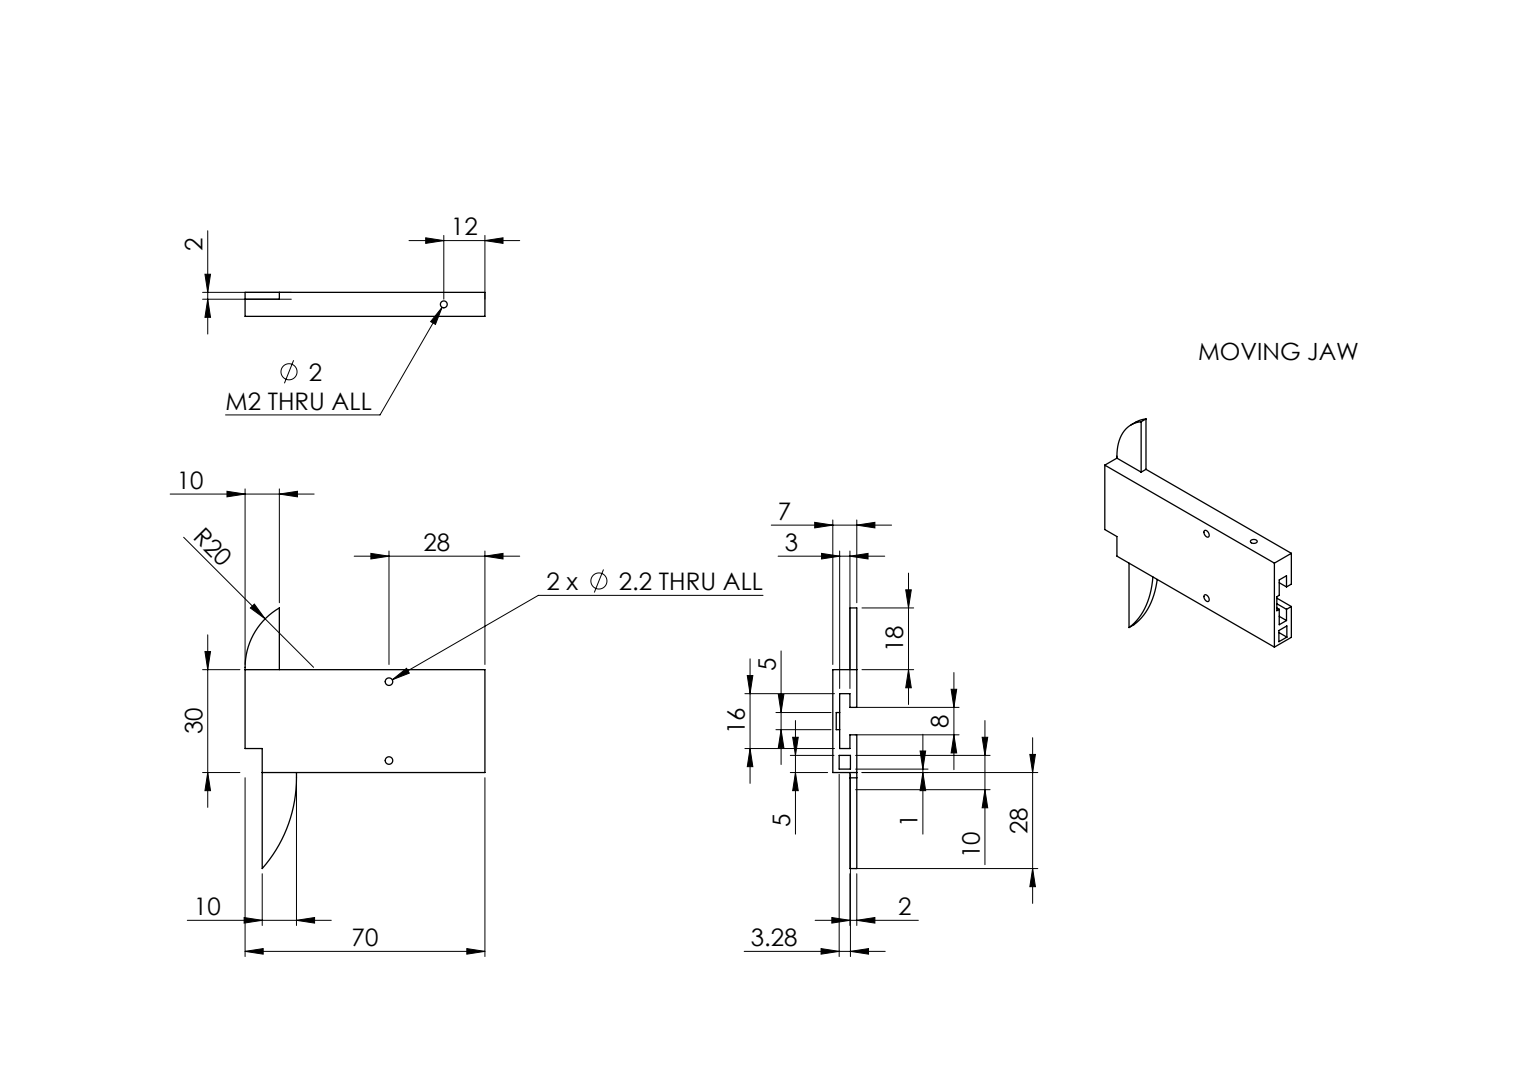
ISO-10303-21;
HEADER;
FILE_DESCRIPTION (('STEP AP214'),
    '1' );
FILE_NAME ('moving jaw.step',
    '2026-10-27T04:40:18',
    ( '' ),
    ( '' ),
    'SwSTEP 2.0',
    'SolidWorks 2026',
    '' );
FILE_SCHEMA (( 'AUTOMOTIVE_DESIGN' ));
ENDSEC;

DATA;
#1=CARTESIAN_POINT ( 'NONE',  ( -49.99998799999998766, -10.00000000000001066, -0.1418111474832477736 ) ) ;
#20=ADVANCED_FACE ( 'NONE', ( #3172 ), #5726, .T. ) ;
#29=ORIENTED_EDGE ( 'NONE', *, *, #855, .F. ) ;
#37=AXIS2_PLACEMENT_3D ( 'NONE', #4538, #3831, #10428 ) ;
#40=VERTEX_POINT ( 'NONE', #7517 ) ;
#41=VERTEX_POINT ( 'NONE', #5843 ) ;
#46=ORIENTED_EDGE ( 'NONE', *, *, #9999, .T. ) ;
#48=PRODUCT ( 'moving jaw', 'moving jaw', '', ( #5785 ) ) ;
#83=SHAPE_REPRESENTATION_RELATIONSHIP ( 'NONE' , 'NONE' ,  #2047, #5753 ) ;
#99=ORIENTED_EDGE ( 'NONE', *, *, #1134, .T. ) ;
#111=LINE ( 'NONE', #735, #8321 ) ;
#115=EDGE_LOOP ( 'NONE', ( #2530, #9133, #537, #4365 ) ) ;
#118=EDGE_CURVE ( 'NONE', #7049, #4198, #6685, .T. ) ;
#125=AXIS2_PLACEMENT_3D ( 'NONE', #8648, #2761, #6933 ) ;
#134=ORIENTED_EDGE ( 'NONE', *, *, #6586, .T. ) ;
#137=FILL_AREA_STYLE ('',( #1868 ) ) ;
#141=EDGE_CURVE ( 'NONE', #5618, #1714, #3939, .T. ) ;
#152=PLANE ( 'NONE',  #5103 ) ;
#159=ORIENTED_EDGE ( 'NONE', *, *, #10440, .T. ) ;
#171=CARTESIAN_POINT ( 'NONE',  ( -77.99999999999998579, 11.49999999999999645, 4.999999999999999112 ) ) ;
#187=CARTESIAN_POINT ( 'NONE',  ( -120.0000000000000000, -4.000000000000019540, -2.000000000000000000 ) ) ;
#201=LINE ( 'NONE', #377, #2655 ) ;
#205=ORIENTED_EDGE ( 'NONE', *, *, #5925, .T. ) ;
#208=LINE ( 'NONE', #3594, #2451 ) ;
#211=VERTEX_POINT ( 'NONE', #6639 ) ;
#214=VECTOR ( 'NONE', #3123, 1000.000000000000000 ) ;
#220=DIRECTION ( 'NONE',  ( -1.000000000000000000, -3.469446951953572774E-16, 0.000000000000000000 ) ) ;
#238=ORIENTED_EDGE ( 'NONE', *, *, #10620, .F. ) ;
#256=( NAMED_UNIT ( * ) SI_UNIT ( $, .STERADIAN. ) SOLID_ANGLE_UNIT ( ) );
#285=FACE_BOUND ( 'NONE', #5927, .T. ) ;
#299=FACE_BOUND ( 'NONE', #9767, .T. ) ;
#306=ORIENTED_EDGE ( 'NONE', *, *, #5403, .T. ) ;
#310=PLANE ( 'NONE',  #5287 ) ;
#324=DIRECTION ( 'NONE',  ( 1.000000000000000000, 2.478176394252581387E-17, 0.000000000000000000 ) ) ;
#330=CARTESIAN_POINT ( 'NONE',  ( -49.99998799999998766, -10.00000000000001066, 5.282956808509874826E-15 ) ) ;
#346=AXIS2_PLACEMENT_3D ( 'NONE', #4920, #5760, #10085 ) ;
#372=DIRECTION ( 'NONE',  ( -1.000000000000000000, 0.000000000000000000, 0.000000000000000000 ) ) ;
#377=CARTESIAN_POINT ( 'NONE',  ( -114.9999999999999289, -7.999999999999998224, -2.000000000000000000 ) ) ;
#378=CYLINDRICAL_SURFACE ( 'NONE', #125, 1.000000000000000888 ) ;
#392=DIRECTION ( 'NONE',  ( 0.000000000000000000, 5.282956808509869699E-16, 1.000000000000000000 ) ) ;
#408=FACE_OUTER_BOUND ( 'NONE', #9322, .T. ) ;
#412=EDGE_CURVE ( 'NONE', #7538, #2208, #10852, .T. ) ;
#417=ORIENTED_EDGE ( 'NONE', *, *, #855, .T. ) ;
#425=AXIS2_PLACEMENT_3D ( 'NONE', #5057, #4070, #1572 ) ;
#426=DIRECTION ( 'NONE',  ( 0.000000000000000000, -0.000000000000000000, -1.000000000000000000 ) ) ;
#430=CARTESIAN_POINT ( 'NONE',  ( -104.9999999999999289, -16.54248688935409106, -2.000000000000000000 ) ) ;
#433=AXIS2_PLACEMENT_3D ( 'NONE', #10103, #729, #1616 ) ;
#448=ORIENTED_EDGE ( 'NONE', *, *, #4377, .F. ) ;
#451=CARTESIAN_POINT ( 'NONE',  ( -49.99999999999998579, -8.000000000000000000, 0.000000000000000000 ) ) ;
#454=DIRECTION ( 'NONE',  ( 1.000000000000000000, 0.000000000000000000, 0.000000000000000000 ) ) ;
#457=CARTESIAN_POINT ( 'NONE',  ( -49.99999999999998579, -2.500000000000000444, 83.15773105863907233 ) ) ;
#460=DIRECTION ( 'NONE',  ( -1.000000000000000000, 0.000000000000000000, 0.000000000000000000 ) ) ;
#462=CARTESIAN_POINT ( 'NONE',  ( -105.0000000000000000, 2.500000000000000000, 3.000000000000000000 ) ) ;
#464=EDGE_LOOP ( 'NONE', ( #3656, #644 ) ) ;
#489=ORIENTED_EDGE ( 'NONE', *, *, #8078, .F. ) ;
#498=LINE ( 'NONE', #8221, #3700 ) ;
#505=VECTOR ( 'NONE', #9411, 1000.000000000000000 ) ;
#512=DIRECTION ( 'NONE',  ( 0.000000000000000000, 1.000000000000000000, 0.000000000000000000 ) ) ;
#518=LINE ( 'NONE', #6516, #873 ) ;
#527=ORIENTED_EDGE ( 'NONE', *, *, #2808, .T. ) ;
#528=CARTESIAN_POINT ( 'NONE',  ( -120.0000000000000000, -4.000000000000019540, 0.000000000000000000 ) ) ;
#536=CIRCLE ( 'NONE', #1421, 40.00000000000000711 ) ;
#537=ORIENTED_EDGE ( 'NONE', *, *, #9340, .T. ) ;
#544=VERTEX_POINT ( 'NONE', #3013 ) ;
#551=VECTOR ( 'NONE', #1388, 1000.000000000000000 ) ;
#558=DIRECTION ( 'NONE',  ( -0.000000000000000000, -0.000000000000000000, -1.000000000000000000 ) ) ;
#566=DIRECTION ( 'NONE',  ( -1.000000000000000000, 0.000000000000000000, 0.000000000000000000 ) ) ;
#570=VERTEX_POINT ( 'NONE', #3901 ) ;
#571=LINE ( 'NONE', #7345, #5302 ) ;
#572=EDGE_CURVE ( 'NONE', #10486, #930, #1997, .T. ) ;
#574=ORIENTED_EDGE ( 'NONE', *, *, #8698, .F. ) ;
#595=CARTESIAN_POINT ( 'NONE',  ( 0.000000000000000000, 0.000000000000000000, 0.000000000000000000 ) ) ;
#596=ORIENTED_EDGE ( 'NONE', *, *, #6504, .F. ) ;
#610=VECTOR ( 'NONE', #6030, 1000.000000000000000 ) ;
#611=CYLINDRICAL_SURFACE ( 'NONE', #4223, 1.099999999999989875 ) ;
#616=CARTESIAN_POINT ( 'NONE',  ( -144.9999999999999147, -16.54248688935410883, -2.000000000000000000 ) ) ;
#624=EDGE_LOOP ( 'NONE', ( #4577, #6804, #1440, #7145 ) ) ;
#631=DIRECTION ( 'NONE',  ( 0.000000000000000000, 0.000000000000000000, -1.000000000000000000 ) ) ;
#639=FACE_OUTER_BOUND ( 'NONE', #8188, .T. ) ;
#643=DIRECTION ( 'NONE',  ( 0.000000000000000000, 0.000000000000000000, -1.000000000000000000 ) ) ;
#644=ORIENTED_EDGE ( 'NONE', *, *, #9959, .F. ) ;
#655=EDGE_LOOP ( 'NONE', ( #7806, #6596, #6590, #7819, #2641, #6040 ) ) ;
#657=EDGE_CURVE ( 'NONE', #5688, #8551, #9953, .T. ) ;
#672=CARTESIAN_POINT ( 'NONE',  ( -76.89999999999999147, -11.50000000000000711, -2.000000000000001332 ) ) ;
#673=DIRECTION ( 'NONE',  ( -3.469446951953572774E-16, 1.000000000000000000, 0.000000000000000000 ) ) ;
#685=ORIENTED_EDGE ( 'NONE', *, *, #10440, .F. ) ;
#699=VECTOR ( 'NONE', #786, 1000.000000000000000 ) ;
#710=VECTOR ( 'NONE', #6574, 1000.000000000000000 ) ;
#716=FACE_OUTER_BOUND ( 'NONE', #7545, .T. ) ;
#719=LINE ( 'NONE', #7497, #9735 ) ;
#726=ORIENTED_EDGE ( 'NONE', *, *, #10589, .F. ) ;
#729=DIRECTION ( 'NONE',  ( 0.000000000000000000, -1.000000000000000000, 0.000000000000000000 ) ) ;
#734=CARTESIAN_POINT ( 'NONE',  ( -120.0000000000000000, 3.999999999999980904, -2.000000000000000000 ) ) ;
#735=CARTESIAN_POINT ( 'NONE',  ( -79.09999999999998010, -11.50000000000000711, -2.000000000000000000 ) ) ;
#761=DIRECTION ( 'NONE',  ( -0.000000000000000000, -0.000000000000000000, 1.000000000000000000 ) ) ;
#785=DIRECTION ( 'NONE',  ( 3.965082230804130220E-16, -1.000000000000000000, -0.000000000000000000 ) ) ;
#786=DIRECTION ( 'NONE',  ( 1.110223024625156540E-15, -1.000000000000000000, -0.000000000000000000 ) ) ;
#795=EDGE_CURVE ( 'NONE', #10821, #9418, #1827, .T. ) ;
#808=LINE ( 'NONE', #4293, #610 ) ;
#824=ORIENTED_EDGE ( 'NONE', *, *, #8252, .F. ) ;
#826=EDGE_CURVE ( 'NONE', #1612, #7049, #10099, .T. ) ;
#851=EDGE_CURVE ( 'NONE', #8859, #6858, #8491, .T. ) ;
#853=CARTESIAN_POINT ( 'NONE',  ( 0.000000000000000000, 2.500000000000000000, 3.000000000000000000 ) ) ;
#855=EDGE_CURVE ( 'NONE', #8551, #10821, #6065, .T. ) ;
#856=VECTOR ( 'NONE', #4422, 1000.000000000000000 ) ;
#859=DIRECTION ( 'NONE',  ( -0.000000000000000000, -0.000000000000000000, -1.000000000000000000 ) ) ;
#862=VECTOR ( 'NONE', #785, 1000.000000000000000 ) ;
#863=ORIENTED_EDGE ( 'NONE', *, *, #9461, .F. ) ;
#865=ORIENTED_EDGE ( 'NONE', *, *, #10184, .F. ) ;
#870=ORIENTED_EDGE ( 'NONE', *, *, #9959, .T. ) ;
#873=VECTOR ( 'NONE', #2385, 1000.000000000000000 ) ;
#877=EDGE_LOOP ( 'NONE', ( #7744, #7640, #7709, #8703, #6978 ) ) ;
#880=ORIENTED_EDGE ( 'NONE', *, *, #964, .F. ) ;
#888=LINE ( 'NONE', #4120, #699 ) ;
#892=CARTESIAN_POINT ( 'NONE',  ( -114.9999999999999289, -7.999999999999998224, 0.000000000000000000 ) ) ;
#914=AXIS2_PLACEMENT_3D ( 'NONE', #7457, #10834, #3218 ) ;
#917=LINE ( 'NONE', #10976, #7086 ) ;
#924=ADVANCED_FACE ( 'NONE', ( #6277 ), #5310, .T. ) ;
#930=VERTEX_POINT ( 'NONE', #6996 ) ;
#960=EDGE_CURVE ( 'NONE', #5520, #211, #7167, .T. ) ;
#964=EDGE_CURVE ( 'NONE', #4466, #8509, #4114, .T. ) ;
#974=CARTESIAN_POINT ( 'NONE',  ( -61.99999999999998579, 14.99999999999998579, 0.5000000000000013323 ) ) ;
#985=EDGE_CURVE ( 'NONE', #4938, #4740, #10490, .T. ) ;
#994=DIRECTION ( 'NONE',  ( 1.000000000000000000, 0.000000000000000000, 0.000000000000000000 ) ) ;
#995=FACE_OUTER_BOUND ( 'NONE', #3796, .T. ) ;
#1027=EDGE_LOOP ( 'NONE', ( #8715, #10682 ) ) ;
#1029=AXIS2_PLACEMENT_3D ( 'NONE', #1383, #4866, #8270 ) ;
#1030=CARTESIAN_POINT ( 'NONE',  ( -109.9999999999999574, 14.99999999999998579, 83.15773105863907233 ) ) ;
#1042=ORIENTED_EDGE ( 'NONE', *, *, #6230, .T. ) ;
#1043=CARTESIAN_POINT ( 'NONE',  ( -49.99999999999998579, 14.99999999999998579, 5.000000000000004441 ) ) ;
#1053=DIRECTION ( 'NONE',  ( -1.000000000000000000, 0.000000000000000000, 0.000000000000000000 ) ) ;
#1080=DIRECTION ( 'NONE',  ( 0.000000000000000000, 1.000000000000000000, 0.000000000000000000 ) ) ;
#1082=FACE_OUTER_BOUND ( 'NONE', #624, .T. ) ;
#1092=ORIENTED_EDGE ( 'NONE', *, *, #9052, .T. ) ;
#1100=EDGE_CURVE ( 'NONE', #3973, #7049, #9351, .T. ) ;
#1107=ADVANCED_FACE ( 'NONE', ( #10181 ), #10074, .F. ) ;
#1112=AXIS2_PLACEMENT_3D ( 'NONE', #9864, #10749, #426 ) ;
#1120=DIRECTION ( 'NONE',  ( -1.000000000000000000, 0.000000000000000000, 0.000000000000000000 ) ) ;
#1134=EDGE_CURVE ( 'NONE', #7831, #4618, #1812, .T. ) ;
#1135=CARTESIAN_POINT ( 'NONE',  ( -105.0000000000000000, -2.500000000000000000, 4.000000000000000000 ) ) ;
#1145=PRESENTATION_STYLE_ASSIGNMENT (( #3639 ) ) ;
#1163=PLANE ( 'NONE',  #7675 ) ;
#1165=DIRECTION ( 'NONE',  ( -1.000000000000000000, 0.000000000000000000, -0.000000000000000000 ) ) ;
#1172=CARTESIAN_POINT ( 'NONE',  ( -61.99999999999998579, 14.99999999999998579, 2.500000000000003109 ) ) ;
#1206=( GEOMETRIC_REPRESENTATION_CONTEXT ( 3 ) GLOBAL_UNCERTAINTY_ASSIGNED_CONTEXT ( ( #10045 ) ) GLOBAL_UNIT_ASSIGNED_CONTEXT ( ( #6328, #8215, #10032 ) ) REPRESENTATION_CONTEXT ( 'NONE', 'WORKASPACE' ) );
#1214=VECTOR ( 'NONE', #9599, 1000.000000000000000 ) ;
#1230=CARTESIAN_POINT ( 'NONE',  ( -149.9999999999999716, 8.000000000000000000, 3.000000000000000000 ) ) ;
#1234=EDGE_LOOP ( 'NONE', ( #6576, #8997, #7608, #685, #8217, #3108 ) ) ;
#1250=AXIS2_PLACEMENT_3D ( 'NONE', #6279, #1542, #9834 ) ;
#1252=DIRECTION ( 'NONE',  ( -1.000000000000000000, 0.000000000000000000, -0.000000000000000000 ) ) ;
#1275=FACE_OUTER_BOUND ( 'NONE', #6489, .T. ) ;
#1285=LINE ( 'NONE', #8070, #10882 ) ;
#1286=DIRECTION ( 'NONE',  ( 1.000000000000000000, 0.000000000000000000, 0.000000000000000000 ) ) ;
#1296=VERTEX_POINT ( 'NONE', #1135 ) ;
#1297=CARTESIAN_POINT ( 'NONE',  ( -77.99999999999998579, -11.50000000000000711, 4.999999999999999112 ) ) ;
#1314=AXIS2_PLACEMENT_3D ( 'NONE', #8865, #8146, #1252 ) ;
#1340=EDGE_LOOP ( 'NONE', ( #238, #5363, #5092, #7261, #4256, #4767, #7735, #1853 ) ) ;
#1355=DIRECTION ( 'NONE',  ( -0.000000000000000000, -0.000000000000000000, 1.000000000000000000 ) ) ;
#1356=FACE_BOUND ( 'NONE', #8492, .T. ) ;
#1357=ORIENTED_EDGE ( 'NONE', *, *, #8744, .F. ) ;
#1362=ORIENTED_EDGE ( 'NONE', *, *, #2808, .F. ) ;
#1370=EDGE_LOOP ( 'NONE', ( #6623, #417, #8003, #8924 ) ) ;
#1380=CARTESIAN_POINT ( 'NONE',  ( -119.9999999999999858, 15.67949192431120053, 0.000000000000000000 ) ) ;
#1383=CARTESIAN_POINT ( 'NONE',  ( -77.99999999999998579, 11.49999999999999645, 4.999999999999999112 ) ) ;
#1388=DIRECTION ( 'NONE',  ( -0.000000000000000000, 1.000000000000000000, -0.000000000000000000 ) ) ;
#1404=AXIS2_PLACEMENT_3D ( 'NONE', #1447, #3009, #5714 ) ;
#1408=ADVANCED_FACE ( 'NONE', ( #3035, #5581 ), #9694, .F. ) ;
#1410=CARTESIAN_POINT ( 'NONE',  ( -120.0000000000000000, -8.000000000000000000, -2.000000000000000000 ) ) ;
#1412=DIRECTION ( 'NONE',  ( -1.000000000000000000, 0.000000000000000000, -0.000000000000000000 ) ) ;
#1415=DIRECTION ( 'NONE',  ( -1.000000000000000000, -0.000000000000000000, -0.000000000000000000 ) ) ;
#1417=CARTESIAN_POINT ( 'NONE',  ( -109.9999999999999574, 14.99999999999998579, -2.000000000000000000 ) ) ;
#1421=AXIS2_PLACEMENT_3D ( 'NONE', #4124, #10850, #4069 ) ;
#1440=ORIENTED_EDGE ( 'NONE', *, *, #5121, .T. ) ;
#1442=ORIENTED_EDGE ( 'NONE', *, *, #8241, .F. ) ;
#1447=CARTESIAN_POINT ( 'NONE',  ( -77.99999999999998579, 11.49999999999999645, -2.000000000000001332 ) ) ;
#1452=VERTEX_POINT ( 'NONE', #9917 ) ;
#1459=CARTESIAN_POINT ( 'NONE',  ( -49.99999999999998579, -15.00000000000001243, 5.000000000000004441 ) ) ;
#1469=LINE ( 'NONE', #9130, #2120 ) ;
#1474=VECTOR ( 'NONE', #2291, 1000.000000000000000 ) ;
#1481=DIRECTION ( 'NONE',  ( -3.965082230804130220E-16, 1.000000000000000000, 0.000000000000000000 ) ) ;
#1490=DIRECTION ( 'NONE',  ( -0.000000000000000000, -0.000000000000000000, -1.000000000000000000 ) ) ;
#1495=EDGE_CURVE ( 'NONE', #3366, #2273, #2351, .T. ) ;
#1499=CARTESIAN_POINT ( 'NONE',  ( -49.99999999999998579, 2.500000000000000000, 4.000000000000000000 ) ) ;
#1500=DIRECTION ( 'NONE',  ( -0.000000000000000000, -0.000000000000000000, -1.000000000000000000 ) ) ;
#1501=CARTESIAN_POINT ( 'NONE',  ( -149.9999999999999716, -8.000000000000000000, 3.000000000000000000 ) ) ;
#1509=CARTESIAN_POINT ( 'NONE',  ( -114.9999999999999289, -15.00000000000001421, 5.000000000000004441 ) ) ;
#1519=ADVANCED_FACE ( 'NONE', ( #639 ), #5792, .F. ) ;
#1542=DIRECTION ( 'NONE',  ( 0.000000000000000000, -1.000000000000000000, 0.000000000000000000 ) ) ;
#1563=VECTOR ( 'NONE', #3177, 1000.000000000000000 ) ;
#1565=DIRECTION ( 'NONE',  ( 1.000000000000000000, -0.000000000000000000, 0.000000000000000000 ) ) ;
#1566=CARTESIAN_POINT ( 'NONE',  ( -114.9999999999999289, -15.00000000000001421, 0.000000000000000000 ) ) ;
#1572=DIRECTION ( 'NONE',  ( 0.000000000000000000, 0.000000000000000000, 1.000000000000000000 ) ) ;
#1577=DIRECTION ( 'NONE',  ( -1.000000000000000000, -3.469446951953572774E-16, 0.000000000000000000 ) ) ;
#1583=DIRECTION ( 'NONE',  ( -1.000000000000000000, 0.000000000000000000, -0.000000000000000000 ) ) ;
#1595=CARTESIAN_POINT ( 'NONE',  ( -114.9999999999999147, -43.00000000000000000, -2.000000000000000000 ) ) ;
#1599=VERTEX_POINT ( 'NONE', #2455 ) ;
#1602=ORIENTED_EDGE ( 'NONE', *, *, #118, .T. ) ;
#1612=VERTEX_POINT ( 'NONE', #4125 ) ;
#1616=DIRECTION ( 'NONE',  ( 0.000000000000000000, 0.000000000000000000, -1.000000000000000000 ) ) ;
#1622=DIRECTION ( 'NONE',  ( 0.000000000000000000, -0.000000000000000000, -1.000000000000000000 ) ) ;
#1623=AXIS2_PLACEMENT_3D ( 'NONE', #9057, #2172, #7494 ) ;
#1644=EDGE_CURVE ( 'NONE', #3802, #570, #6077, .T. ) ;
#1650=AXIS2_PLACEMENT_3D ( 'NONE', #595, #643, #7419 ) ;
#1652=DIRECTION ( 'NONE',  ( 0.000000000000000000, 0.000000000000000000, 1.000000000000000000 ) ) ;
#1657=CARTESIAN_POINT ( 'NONE',  ( -49.99998799999998766, -10.00000000000000888, 3.141811147483251965 ) ) ;
#1664=VECTOR ( 'NONE', #4606, 1000.000000000000000 ) ;
#1694=EDGE_CURVE ( 'NONE', #1612, #1296, #8738, .T. ) ;
#1698=VERTEX_POINT ( 'NONE', #8512 ) ;
#1706=DIRECTION ( 'NONE',  ( 1.000000000000000000, 0.000000000000000000, 0.000000000000000000 ) ) ;
#1714=VERTEX_POINT ( 'NONE', #2682 ) ;
#1725=LINE ( 'NONE', #6950, #10974 ) ;
#1748=EDGE_CURVE ( 'NONE', #570, #3802, #2899, .T. ) ;
#1756=LINE ( 'NONE', #7648, #5474 ) ;
#1758=VECTOR ( 'NONE', #994, 1000.000000000000000 ) ;
#1765=STYLED_ITEM ( 'NONE', ( #1145 ), #5753 ) ;
#1790=CARTESIAN_POINT ( 'NONE',  ( -61.99999999999998579, 14.99999999999998579, 1.500000000000002220 ) ) ;
#1812=CIRCLE ( 'NONE', #7492, 1.000000000000000888 ) ;
#1814=ADVANCED_FACE ( 'NONE', ( #1356, #408 ), #3904, .F. ) ;
#1827=LINE ( 'NONE', #5200, #3582 ) ;
#1828=ORIENTED_EDGE ( 'NONE', *, *, #10681, .F. ) ;
#1829=CARTESIAN_POINT ( 'NONE',  ( -114.9999999999999289, -7.999999999999998224, 5.000000000000004441 ) ) ;
#1831=PRODUCT_DEFINITION_SHAPE ( 'NONE', 'NONE',  #3118 ) ;
#1852=CARTESIAN_POINT ( 'NONE',  ( -120.0000000000000000, -8.000000000000000000, -2.000000000000000000 ) ) ;
#1853=ORIENTED_EDGE ( 'NONE', *, *, #6704, .T. ) ;
#1868=FILL_AREA_STYLE_COLOUR ( '', #6571 ) ;
#1872=LINE ( 'NONE', #5243, #5665 ) ;
#1888=CARTESIAN_POINT ( 'NONE',  ( -49.99998799999998766, -14.00000000000001243, -0.1418111474832477736 ) ) ;
#1918=ORIENTED_EDGE ( 'NONE', *, *, #2411, .F. ) ;
#1923=VECTOR ( 'NONE', #9384, 1000.000000000000000 ) ;
#1934=DIRECTION ( 'NONE',  ( 0.000000000000000000, 0.000000000000000000, -1.000000000000000000 ) ) ;
#1947=CARTESIAN_POINT ( 'NONE',  ( -49.99999999999998579, -14.00000000000001243, -0.1418111474832540464 ) ) ;
#1948=ADVANCED_FACE ( 'NONE', ( #5445 ), #8851, .T. ) ;
#1957=EDGE_LOOP ( 'NONE', ( #596, #5706, #4141, #6991 ) ) ;
#1963=LINE ( 'NONE', #6962, #7655 ) ;
#1970=LINE ( 'NONE', #9577, #10874 ) ;
#1977=EDGE_LOOP ( 'NONE', ( #10642, #6739 ) ) ;
#1987=EDGE_CURVE ( 'NONE', #6146, #3291, #10736, .T. ) ;
#1995=DIRECTION ( 'NONE',  ( 0.000000000000000000, -0.000000000000000000, 1.000000000000000000 ) ) ;
#1997=CIRCLE ( 'NONE', #3066, 1.099999999999989875 ) ;
#2032=ORIENTED_EDGE ( 'NONE', *, *, #5591, .F. ) ;
#2036=ORIENTED_EDGE ( 'NONE', *, *, #4732, .T. ) ;
#2038=CARTESIAN_POINT ( 'NONE',  ( -99.99999999999998579, 15.67949192431120053, -2.000000000000000000 ) ) ;
#2042=EDGE_CURVE ( 'NONE', #10433, #1452, #1970, .T. ) ;
#2044=ORIENTED_EDGE ( 'NONE', *, *, #9484, .T. ) ;
#2047=SHAPE_REPRESENTATION ( 'moving jaw', ( #2307 ), #4948 ) ;
#2053=CARTESIAN_POINT ( 'NONE',  ( -120.0000000000000000, -15.00000000000001421, -2.000000000000000000 ) ) ;
#2054=EDGE_LOOP ( 'NONE', ( #2057, #2218, #8952, #10553 ) ) ;
#2056=EDGE_CURVE ( 'NONE', #3973, #3104, #6857, .T. ) ;
#2057=ORIENTED_EDGE ( 'NONE', *, *, #5007, .F. ) ;
#2061=DIRECTION ( 'NONE',  ( 0.000000000000000000, 1.000000000000000000, 0.000000000000000000 ) ) ;
#2067=DIRECTION ( 'NONE',  ( 0.000000000000000000, -1.000000000000000000, 0.000000000000000000 ) ) ;
#2079=DIRECTION ( 'NONE',  ( -0.000000000000000000, 1.000000000000000000, -0.000000000000000000 ) ) ;
#2090=CARTESIAN_POINT ( 'NONE',  ( -49.99999999999998579, -14.00000000000001243, 3.141811147483255073 ) ) ;
#2091=DIRECTION ( 'NONE',  ( -0.000000000000000000, -0.000000000000000000, -1.000000000000000000 ) ) ;
#2092=ORIENTED_EDGE ( 'NONE', *, *, #9950, .F. ) ;
#2100=EDGE_CURVE ( 'NONE', #4938, #3792, #6020, .T. ) ;
#2109=CARTESIAN_POINT ( 'NONE',  ( -144.9999999999999147, -16.54248688935410883, 0.000000000000000000 ) ) ;
#2110=ORIENTED_EDGE ( 'NONE', *, *, #2887, .F. ) ;
#2120=VECTOR ( 'NONE', #1415, 1000.000000000000000 ) ;
#2140=CARTESIAN_POINT ( 'NONE',  ( -61.99999999999998579, 14.99999999999998579, 1.500000000000002220 ) ) ;
#2171=ORIENTED_EDGE ( 'NONE', *, *, #6545, .T. ) ;
#2172=DIRECTION ( 'NONE',  ( 0.000000000000000000, 0.000000000000000000, -1.000000000000000000 ) ) ;
#2175=DIRECTION ( 'NONE',  ( 0.000000000000000000, 0.000000000000000000, -1.000000000000000000 ) ) ;
#2181=ADVANCED_FACE ( 'NONE', ( #3629 ), #6809, .F. ) ;
#2188=VERTEX_POINT ( 'NONE', #1417 ) ;
#2196=DIRECTION ( 'NONE',  ( 0.000000000000000000, 0.000000000000000000, 1.000000000000000000 ) ) ;
#2204=VERTEX_POINT ( 'NONE', #10463 ) ;
#2208=VERTEX_POINT ( 'NONE', #6251 ) ;
#2210=AXIS2_PLACEMENT_3D ( 'NONE', #2953, #6816, #5073 ) ;
#2218=ORIENTED_EDGE ( 'NONE', *, *, #5229, .F. ) ;
#2233=DIRECTION ( 'NONE',  ( -0.000000000000000000, -0.000000000000000000, -1.000000000000000000 ) ) ;
#2245=PLANE ( 'NONE',  #7427 ) ;
#2248=CARTESIAN_POINT ( 'NONE',  ( -105.0000000000000000, 2.500000000000000000, 4.000000000000000000 ) ) ;
#2258=VERTEX_POINT ( 'NONE', #8094 ) ;
#2273=VERTEX_POINT ( 'NONE', #5629 ) ;
#2275=VECTOR ( 'NONE', #8665, 1000.000000000000000 ) ;
#2283=AXIS2_PLACEMENT_3D ( 'NONE', #8664, #6785, #2501 ) ;
#2291=DIRECTION ( 'NONE',  ( 0.000000000000000000, -1.000000000000000000, 0.000000000000000000 ) ) ;
#2305=LINE ( 'NONE', #3501, #2306 ) ;
#2306=VECTOR ( 'NONE', #7793, 1000.000000000000000 ) ;
#2307=AXIS2_PLACEMENT_3D ( 'NONE', #5193, #3646, #1706 ) ;
#2328=ADVANCED_FACE ( 'NONE', ( #299, #7976 ), #4736, .T. ) ;
#2335=DIRECTION ( 'NONE',  ( -1.000000000000000000, 0.000000000000000000, 0.000000000000000000 ) ) ;
#2341=DIRECTION ( 'NONE',  ( 0.000000000000000000, 0.000000000000000000, -1.000000000000000000 ) ) ;
#2347=FACE_OUTER_BOUND ( 'NONE', #7855, .T. ) ;
#2351=LINE ( 'NONE', #9970, #10146 ) ;
#2352=AXIS2_PLACEMENT_3D ( 'NONE', #10029, #5915, #1583 ) ;
#2366=DIRECTION ( 'NONE',  ( -1.000000000000000000, 0.000000000000000000, 0.000000000000000000 ) ) ;
#2374=ORIENTED_EDGE ( 'NONE', *, *, #5254, .T. ) ;
#2376=VERTEX_POINT ( 'NONE', #672 ) ;
#2379=LINE ( 'NONE', #7496, #9200 ) ;
#2385=DIRECTION ( 'NONE',  ( -0.000000000000000000, -0.000000000000000000, 1.000000000000000000 ) ) ;
#2391=CARTESIAN_POINT ( 'NONE',  ( -49.99999999999998579, -15.00000000000001243, 5.000000000000004441 ) ) ;
#2399=ORIENTED_EDGE ( 'NONE', *, *, #10843, .T. ) ;
#2401=EDGE_CURVE ( 'NONE', #2572, #8685, #3085, .T. ) ;
#2411=EDGE_CURVE ( 'NONE', #8509, #8229, #4059, .T. ) ;
#2418=LINE ( 'NONE', #8374, #4937 ) ;
#2435=LINE ( 'NONE', #6624, #10095 ) ;
#2451=VECTOR ( 'NONE', #6937, 1000.000000000000000 ) ;
#2452=CARTESIAN_POINT ( 'NONE',  ( -105.0000000000000000, 0.000000000000000000, 3.000000000000000000 ) ) ;
#2455=CARTESIAN_POINT ( 'NONE',  ( -120.0000000000000000, 8.000000000000000000, 0.000000000000000000 ) ) ;
#2472=CARTESIAN_POINT ( 'NONE',  ( -61.99999999999998579, -15.00000000000001421, 1.500000000000002220 ) ) ;
#2484=ORIENTED_EDGE ( 'NONE', *, *, #7252, .T. ) ;
#2501=DIRECTION ( 'NONE',  ( 0.000000000000000000, 0.000000000000000000, 1.000000000000000000 ) ) ;
#2510=DIRECTION ( 'NONE',  ( 0.000000000000000000, -1.000000000000000000, 0.000000000000000000 ) ) ;
#2513=CARTESIAN_POINT ( 'NONE',  ( -61.99999999999998579, 14.99999999999998579, 1.500000000000002220 ) ) ;
#2514=CLOSED_SHELL ( 'NONE', ( #5138, #1519, #6235, #7428, #1408, #1814, #2328, #2854, #2804, #7177, #9480, #8967, #9873, #4092, #4117, #3301, #5550, #1107, #1948, #4029, #5963, #6423, #2784, #6008, #4487, #2181, #4923, #4555, #5342, #5724, #924, #10376, #9047, #2947, #5677, #3237, #20, #3957, #7646, #8158, #8848 ) ) ;
#2519=ORIENTED_EDGE ( 'NONE', *, *, #6829, .T. ) ;
#2529=CARTESIAN_POINT ( 'NONE',  ( -49.99999999999998579, -14.00000000000001243, 83.15773105863907233 ) ) ;
#2530=ORIENTED_EDGE ( 'NONE', *, *, #985, .T. ) ;
#2541=ORIENTED_EDGE ( 'NONE', *, *, #10681, .T. ) ;
#2550=DIRECTION ( 'NONE',  ( -0.000000000000000000, -0.000000000000000000, -1.000000000000000000 ) ) ;
#2560=CARTESIAN_POINT ( 'NONE',  ( -49.99999999999998579, -15.00000000000001243, 4.000000000000003553 ) ) ;
#2571=CARTESIAN_POINT ( 'NONE',  ( -61.99999999999998579, 14.99999999999998579, 0.5000000000000013323 ) ) ;
#2572=VERTEX_POINT ( 'NONE', #4262 ) ;
#2587=EDGE_CURVE ( 'NONE', #9263, #2273, #6891, .T. ) ;
#2625=ORIENTED_EDGE ( 'NONE', *, *, #2056, .T. ) ;
#2639=LINE ( 'NONE', #6025, #505 ) ;
#2641=ORIENTED_EDGE ( 'NONE', *, *, #6974, .F. ) ;
#2650=ORIENTED_EDGE ( 'NONE', *, *, #9461, .T. ) ;
#2655=VECTOR ( 'NONE', #8770, 1000.000000000000000 ) ;
#2665=ORIENTED_EDGE ( 'NONE', *, *, #9052, .F. ) ;
#2676=LINE ( 'NONE', #5212, #1758 ) ;
#2682=CARTESIAN_POINT ( 'NONE',  ( -61.99999999999998579, -8.000000000000000000, 0.5000000000000013323 ) ) ;
#2693=EDGE_CURVE ( 'NONE', #4361, #5520, #1285, .T. ) ;
#2705=LINE ( 'NONE', #974, #3898 ) ;
#2707=VECTOR ( 'NONE', #10392, 1000.000000000000000 ) ;
#2726=LINE ( 'NONE', #4435, #7598 ) ;
#2747=DIRECTION ( 'NONE',  ( -1.000000000000000000, -0.000000000000000000, -0.000000000000000000 ) ) ;
#2761=DIRECTION ( 'NONE',  ( -0.000000000000000000, 1.000000000000000000, -0.000000000000000000 ) ) ;
#2765=EDGE_LOOP ( 'NONE', ( #10564, #10658, #6014, #824 ) ) ;
#2774=ORIENTED_EDGE ( 'NONE', *, *, #412, .T. ) ;
#2782=DIRECTION ( 'NONE',  ( 0.000000000000000000, 0.000000000000000000, -1.000000000000000000 ) ) ;
#2784=ADVANCED_FACE ( 'NONE', ( #3780 ), #7228, .T. ) ;
#2788=CARTESIAN_POINT ( 'NONE',  ( 0.000000000000000000, 0.000000000000000000, 5.000000000000000000 ) ) ;
#2804=ADVANCED_FACE ( 'NONE', ( #4714 ), #3062, .F. ) ;
#2808=EDGE_CURVE ( 'NONE', #2208, #10486, #3720, .T. ) ;
#2826=ORIENTED_EDGE ( 'NONE', *, *, #9859, .F. ) ;
#2829=CARTESIAN_POINT ( 'NONE',  ( -49.99999999999998579, 8.000000000000001776, 83.15773105863907233 ) ) ;
#2840=AXIS2_PLACEMENT_3D ( 'NONE', #2788, #7066, #5389 ) ;
#2854=ADVANCED_FACE ( 'NONE', ( #6459, #5607 ), #8177, .F. ) ;
#2865=ORIENTED_EDGE ( 'NONE', *, *, #5787, .F. ) ;
#2884=AXIS2_PLACEMENT_3D ( 'NONE', #4167, #4122, #6532 ) ;
#2887=EDGE_CURVE ( 'NONE', #1698, #2376, #4857, .T. ) ;
#2897=FACE_OUTER_BOUND ( 'NONE', #3419, .T. ) ;
#2899=CIRCLE ( 'NONE', #9104, 1.000000000000000888 ) ;
#2904=PLANE ( 'NONE',  #9212 ) ;
#2907=ORIENTED_EDGE ( 'NONE', *, *, #9894, .T. ) ;
#2925=EDGE_CURVE ( 'NONE', #9418, #5688, #808, .T. ) ;
#2935=DIRECTION ( 'NONE',  ( -0.000000000000000000, -1.000000000000000000, -0.000000000000000000 ) ) ;
#2947=ADVANCED_FACE ( 'NONE', ( #5921 ), #9307, .F. ) ;
#2953=CARTESIAN_POINT ( 'NONE',  ( -120.0000000000000000, -15.00000000000001421, 83.15773105863907233 ) ) ;
#2988=CARTESIAN_POINT ( 'NONE',  ( 0.000000000000000000, -2.500000000000000000, 3.000000000000000000 ) ) ;
#2991=AXIS2_PLACEMENT_3D ( 'NONE', #2140, #2079, #2196 ) ;
#2999=CIRCLE ( 'NONE', #1404, 1.099999999999989875 ) ;
#3009=DIRECTION ( 'NONE',  ( -0.000000000000000000, -0.000000000000000000, -1.000000000000000000 ) ) ;
#3013=CARTESIAN_POINT ( 'NONE',  ( -49.99999999999998579, -2.500000000000000000, 3.000000000000000000 ) ) ;
#3014=ORIENTED_EDGE ( 'NONE', *, *, #10500, .T. ) ;
#3026=ORIENTED_EDGE ( 'NONE', *, *, #1748, .T. ) ;
#3035=FACE_OUTER_BOUND ( 'NONE', #1234, .T. ) ;
#3062=PLANE ( 'NONE',  #6813 ) ;
#3066=AXIS2_PLACEMENT_3D ( 'NONE', #5324, #2233, #2335 ) ;
#3070=LINE ( 'NONE', #9849, #4080 ) ;
#3073=DIRECTION ( 'NONE',  ( -1.000000000000000000, 0.000000000000000000, 0.000000000000000000 ) ) ;
#3081=PLANE ( 'NONE',  #6384 ) ;
#3085=CIRCLE ( 'NONE', #433, 1.000000000000000888 ) ;
#3095=FACE_OUTER_BOUND ( 'NONE', #10378, .T. ) ;
#3100=ORIENTED_EDGE ( 'NONE', *, *, #5058, .F. ) ;
#3104=VERTEX_POINT ( 'NONE', #1499 ) ;
#3108=ORIENTED_EDGE ( 'NONE', *, *, #5529, .T. ) ;
#3118=PRODUCT_DEFINITION ( 'UNKNOWN', '', #7460, #8348 ) ;
#3120=CARTESIAN_POINT ( 'NONE',  ( -49.99999999999998579, 8.000000000000000000, 3.000000000000000000 ) ) ;
#3123=DIRECTION ( 'NONE',  ( 0.000000000000000000, 0.000000000000000000, -1.000000000000000000 ) ) ;
#3141=CARTESIAN_POINT ( 'NONE',  ( -114.9999999999999289, -7.999999999999998224, -2.000000000000000000 ) ) ;
#3152=VERTEX_POINT ( 'NONE', #6199 ) ;
#3157=LINE ( 'NONE', #8320, #551 ) ;
#3167=EDGE_CURVE ( 'NONE', #8229, #5900, #9987, .T. ) ;
#3172=FACE_OUTER_BOUND ( 'NONE', #10185, .T. ) ;
#3177=DIRECTION ( 'NONE',  ( 1.000000000000000000, 0.000000000000000000, 0.000000000000000000 ) ) ;
#3209=ORIENTED_EDGE ( 'NONE', *, *, #5754, .T. ) ;
#3218=DIRECTION ( 'NONE',  ( 1.000000000000000000, 0.000000000000000000, -0.000000000000000000 ) ) ;
#3224=FACE_BOUND ( 'NONE', #1027, .T. ) ;
#3232=ORIENTED_EDGE ( 'NONE', *, *, #7753, .F. ) ;
#3237=ADVANCED_FACE ( 'NONE', ( #4579 ), #5237, .T. ) ;
#3257=ORIENTED_EDGE ( 'NONE', *, *, #5403, .F. ) ;
#3262=ORIENTED_EDGE ( 'NONE', *, *, #7252, .F. ) ;
#3284=CYLINDRICAL_SURFACE ( 'NONE', #7591, 1.099999999999989875 ) ;
#3291=VERTEX_POINT ( 'NONE', #4026 ) ;
#3297=CARTESIAN_POINT ( 'NONE',  ( -61.99999999999998579, -15.00000000000001421, 2.500000000000003109 ) ) ;
#3301=ADVANCED_FACE ( 'NONE', ( #3095 ), #9817, .T. ) ;
#3366=VERTEX_POINT ( 'NONE', #4907 ) ;
#3375=DIRECTION ( 'NONE',  ( -0.000000000000000000, -0.000000000000000000, -1.000000000000000000 ) ) ;
#3377=FACE_OUTER_BOUND ( 'NONE', #9807, .T. ) ;
#3396=ORIENTED_EDGE ( 'NONE', *, *, #1100, .T. ) ;
#3419=EDGE_LOOP ( 'NONE', ( #2541, #10410, #7823, #7330 ) ) ;
#3421=DIRECTION ( 'NONE',  ( -1.000000000000000000, 0.000000000000000000, 0.000000000000000000 ) ) ;
#3431=VERTEX_POINT ( 'NONE', #9295 ) ;
#3443=DIRECTION ( 'NONE',  ( -0.000000000000000000, -0.000000000000000000, 1.000000000000000000 ) ) ;
#3484=ORIENTED_EDGE ( 'NONE', *, *, #5576, .F. ) ;
#3495=LINE ( 'NONE', #8616, #6560 ) ;
#3501=CARTESIAN_POINT ( 'NONE',  ( -120.0000000000000000, 8.000000000000000000, 83.15773105863907233 ) ) ;
#3515=ORIENTED_EDGE ( 'NONE', *, *, #1495, .T. ) ;
#3523=ORIENTED_EDGE ( 'NONE', *, *, #9098, .T. ) ;
#3527=DIRECTION ( 'NONE',  ( -0.000000000000000000, -0.000000000000000000, -1.000000000000000000 ) ) ;
#3531=CIRCLE ( 'NONE', #10263, 1.000000000000000888 ) ;
#3558=CARTESIAN_POINT ( 'NONE',  ( -114.9999999999999289, -7.999999999999998224, -2.000000000000000000 ) ) ;
#3582=VECTOR ( 'NONE', #8437, 1000.000000000000000 ) ;
#3585=VERTEX_POINT ( 'NONE', #1509 ) ;
#3586=CARTESIAN_POINT ( 'NONE',  ( -61.99999999999998579, -15.00000000000001421, 1.500000000000002220 ) ) ;
#3592=EDGE_CURVE ( 'NONE', #9418, #5520, #6577, .T. ) ;
#3594=CARTESIAN_POINT ( 'NONE',  ( -120.0000000000000000, 3.999999999999980904, -2.000000000000000000 ) ) ;
#3607=EDGE_CURVE ( 'NONE', #2376, #1698, #4827, .T. ) ;
#3608=CARTESIAN_POINT ( 'NONE',  ( -104.9999999999999147, -15.00000000000001421, 0.000000000000000000 ) ) ;
#3617=EDGE_CURVE ( 'NONE', #3964, #8912, #9902, .T. ) ;
#3623=ORIENTED_EDGE ( 'NONE', *, *, #10813, .T. ) ;
#3629=FACE_OUTER_BOUND ( 'NONE', #2765, .T. ) ;
#3639=SURFACE_STYLE_USAGE ( .BOTH. , #6203 ) ;
#3646=DIRECTION ( 'NONE',  ( 0.000000000000000000, 0.000000000000000000, 1.000000000000000000 ) ) ;
#3656=ORIENTED_EDGE ( 'NONE', *, *, #141, .F. ) ;
#3660=CARTESIAN_POINT ( 'NONE',  ( -149.9999999999999716, -8.000000000000000000, 3.000000000000000000 ) ) ;
#3665=DIRECTION ( 'NONE',  ( 0.000000000000000000, -0.000000000000000000, -1.000000000000000000 ) ) ;
#3667=DIRECTION ( 'NONE',  ( -0.000000000000000000, -0.000000000000000000, -1.000000000000000000 ) ) ;
#3669=FACE_OUTER_BOUND ( 'NONE', #655, .T. ) ;
#3676=FACE_OUTER_BOUND ( 'NONE', #1957, .T. ) ;
#3696=AXIS2_PLACEMENT_3D ( 'NONE', #3838, #2175, #10609 ) ;
#3700=VECTOR ( 'NONE', #6450, 1000.000000000000000 ) ;
#3706=EDGE_LOOP ( 'NONE', ( #8583, #4737, #2374, #3623 ) ) ;
#3720=LINE ( 'NONE', #8122, #1664 ) ;
#3729=LINE ( 'NONE', #1172, #10253 ) ;
#3775=DIRECTION ( 'NONE',  ( 1.000000000000000000, -0.000000000000000000, 0.000000000000000000 ) ) ;
#3780=FACE_OUTER_BOUND ( 'NONE', #10079, .T. ) ;
#3783=AXIS2_PLACEMENT_3D ( 'NONE', #2513, #6689, #10851 ) ;
#3788=PLANE ( 'NONE',  #9928 ) ;
#3792=VERTEX_POINT ( 'NONE', #4157 ) ;
#3795=VECTOR ( 'NONE', #4515, 1000.000000000000000 ) ;
#3796=EDGE_LOOP ( 'NONE', ( #2519, #2032, #2907, #2044 ) ) ;
#3802=VERTEX_POINT ( 'NONE', #4366 ) ;
#3831=DIRECTION ( 'NONE',  ( 0.000000000000000000, -0.000000000000000000, 1.000000000000000000 ) ) ;
#3838=CARTESIAN_POINT ( 'NONE',  ( 0.000000000000000000, 0.000000000000000000, 4.000000000000000000 ) ) ;
#3847=UNCERTAINTY_MEASURE_WITH_UNIT (LENGTH_MEASURE( 1.000000000000000082E-05 ), #4408, 'distance_accuracy_value', 'NONE');
#3855=ORIENTED_EDGE ( 'NONE', *, *, #6412, .T. ) ;
#3887=ORIENTED_EDGE ( 'NONE', *, *, #2925, .F. ) ;
#3888=CARTESIAN_POINT ( 'NONE',  ( -49.99999999999998579, -10.00000000000000888, -0.1418111474832519925 ) ) ;
#3890=VECTOR ( 'NONE', #4949, 1000.000000000000000 ) ;
#3898=VECTOR ( 'NONE', #6147, 1000.000000000000000 ) ;
#3901=CARTESIAN_POINT ( 'NONE',  ( -61.99999999999998579, 14.99999999999998579, 2.500000000000003109 ) ) ;
#3904=PLANE ( 'NONE',  #7164 ) ;
#3924=EDGE_LOOP ( 'NONE', ( #9884, #7845, #4646, #7601 ) ) ;
#3933=ORIENTED_EDGE ( 'NONE', *, *, #10027, .T. ) ;
#3936=DIRECTION ( 'NONE',  ( -1.000000000000000000, 0.000000000000000000, 0.000000000000000000 ) ) ;
#3939=CIRCLE ( 'NONE', #2884, 1.000000000000000888 ) ;
#3941=EDGE_LOOP ( 'NONE', ( #5298, #5003, #7576, #5126, #9431, #6674, #5871, #3855 ) ) ;
#3954=LINE ( 'NONE', #8285, #4605 ) ;
#3955=DIRECTION ( 'NONE',  ( -0.000000000000000000, 1.000000000000000000, 0.000000000000000000 ) ) ;
#3957=ADVANCED_FACE ( 'NONE', ( #5257 ), #1163, .F. ) ;
#3964=VERTEX_POINT ( 'NONE', #1043 ) ;
#3969=PLANE ( 'NONE',  #5656 ) ;
#3973=VERTEX_POINT ( 'NONE', #9783 ) ;
#3994=VERTEX_POINT ( 'NONE', #451 ) ;
#3998=FACE_OUTER_BOUND ( 'NONE', #3941, .T. ) ;
#4003=DIRECTION ( 'NONE',  ( 3.965082230804130220E-16, -1.000000000000000000, -0.000000000000000000 ) ) ;
#4006=ORIENTED_EDGE ( 'NONE', *, *, #412, .F. ) ;
#4010=LINE ( 'NONE', #9019, #4752 ) ;
#4026=CARTESIAN_POINT ( 'NONE',  ( -120.0000000000000000, 8.000000000000000000, 3.000000000000000000 ) ) ;
#4029=ADVANCED_FACE ( 'NONE', ( #6563 ), #6506, .T. ) ;
#4036=ORIENTED_EDGE ( 'NONE', *, *, #2056, .F. ) ;
#4054=VERTEX_POINT ( 'NONE', #8120 ) ;
#4059=LINE ( 'NONE', #7459, #6627 ) ;
#4069=DIRECTION ( 'NONE',  ( -1.000000000000000000, 0.000000000000000000, 0.000000000000000000 ) ) ;
#4070=DIRECTION ( 'NONE',  ( -0.000000000000000000, 1.000000000000000000, -0.000000000000000000 ) ) ;
#4080=VECTOR ( 'NONE', #4780, 1000.000000000000000 ) ;
#4083=ORIENTED_EDGE ( 'NONE', *, *, #7073, .F. ) ;
#4092=ADVANCED_FACE ( 'NONE', ( #7390 ), #10725, .T. ) ;
#4096=ORIENTED_EDGE ( 'NONE', *, *, #960, .T. ) ;
#4100=DIRECTION ( 'NONE',  ( 0.000000000000000000, -0.000000000000000000, 1.000000000000000000 ) ) ;
#4114=CIRCLE ( 'NONE', #37, 20.00000000000000355 ) ;
#4117=ADVANCED_FACE ( 'NONE', ( #716 ), #10877, .F. ) ;
#4118=CARTESIAN_POINT ( 'NONE',  ( -114.9999999999999147, -43.00000000000000000, -2.000000000000000000 ) ) ;
#4120=CARTESIAN_POINT ( 'NONE',  ( -119.9999999999999716, 8.000000000000001776, 0.000000000000000000 ) ) ;
#4122=DIRECTION ( 'NONE',  ( 0.000000000000000000, 1.000000000000000000, 0.000000000000000000 ) ) ;
#4124=CARTESIAN_POINT ( 'NONE',  ( -144.9999999999999147, -16.54248688935410883, -2.000000000000000000 ) ) ;
#4125=CARTESIAN_POINT ( 'NONE',  ( -105.0000000000000000, 2.500000000000000000, 4.000000000000000000 ) ) ;
#4141=ORIENTED_EDGE ( 'NONE', *, *, #6023, .T. ) ;
#4155=CARTESIAN_POINT ( 'NONE',  ( -120.0000000000000000, 14.99999999999998579, 5.000000000000004441 ) ) ;
#4157=CARTESIAN_POINT ( 'NONE',  ( -120.0000000000000000, -4.000000000000019540, 0.000000000000000000 ) ) ;
#4160=CARTESIAN_POINT ( 'NONE',  ( -120.0000000000000000, -4.000000000000019540, -2.000000000000000000 ) ) ;
#4167=CARTESIAN_POINT ( 'NONE',  ( -61.99999999999998579, -8.000000000000000000, 1.500000000000002220 ) ) ;
#4180=EDGE_LOOP ( 'NONE', ( #1442, #7293, #5341, #7707 ) ) ;
#4193=LINE ( 'NONE', #1657, #7636 ) ;
#4198=VERTEX_POINT ( 'NONE', #7812 ) ;
#4223=AXIS2_PLACEMENT_3D ( 'NONE', #8062, #558, #3936 ) ;
#4236=CARTESIAN_POINT ( 'NONE',  ( -120.0000000000000000, 14.99999999999998579, 5.000000000000004441 ) ) ;
#4250=ORIENTED_EDGE ( 'NONE', *, *, #7867, .F. ) ;
#4256=ORIENTED_EDGE ( 'NONE', *, *, #9844, .F. ) ;
#4262=CARTESIAN_POINT ( 'NONE',  ( -61.99999999999998579, 8.000000000000000000, 2.500000000000003109 ) ) ;
#4293=CARTESIAN_POINT ( 'NONE',  ( -120.0000000000000000, -15.00000000000001421, 0.000000000000000000 ) ) ;
#4300=ORIENTED_EDGE ( 'NONE', *, *, #2587, .F. ) ;
#4308=AXIS2_PLACEMENT_3D ( 'NONE', #8589, #859, #4875 ) ;
#4312=LINE ( 'NONE', #1829, #8513 ) ;
#4337=CARTESIAN_POINT ( 'NONE',  ( 0.000000000000000000, 0.000000000000000000, 0.000000000000000000 ) ) ;
#4347=CARTESIAN_POINT ( 'NONE',  ( -49.99999999999998579, 3.999999999999980904, 0.000000000000000000 ) ) ;
#4361=VERTEX_POINT ( 'NONE', #430 ) ;
#4365=ORIENTED_EDGE ( 'NONE', *, *, #2100, .F. ) ;
#4366=CARTESIAN_POINT ( 'NONE',  ( -61.99999999999998579, 14.99999999999998579, 0.5000000000000013323 ) ) ;
#4374=LINE ( 'NONE', #457, #6002 ) ;
#4377=EDGE_CURVE ( 'NONE', #8566, #7983, #10470, .T. ) ;
#4380=LINE ( 'NONE', #3558, #8498 ) ;
#4393=CARTESIAN_POINT ( 'NONE',  ( -49.99999999999998579, 2.500000000000000444, 83.15773105863907233 ) ) ;
#4408=( LENGTH_UNIT ( ) NAMED_UNIT ( * ) SI_UNIT ( .MILLI., .METRE. ) );
#4416=VECTOR ( 'NONE', #6796, 1000.000000000000000 ) ;
#4422=DIRECTION ( 'NONE',  ( 0.000000000000000000, 1.000000000000000000, 0.000000000000000000 ) ) ;
#4428=ORIENTED_EDGE ( 'NONE', *, *, #7372, .T. ) ;
#4435=CARTESIAN_POINT ( 'NONE',  ( -114.9999999999999289, -7.999999999999998224, -2.000000000000000000 ) ) ;
#4436=LINE ( 'NONE', #5497, #7776 ) ;
#4446=EDGE_CURVE ( 'NONE', #9263, #7983, #6259, .T. ) ;
#4454=VECTOR ( 'NONE', #10396, 1000.000000000000000 ) ;
#4460=ORIENTED_EDGE ( 'NONE', *, *, #1987, .T. ) ;
#4466=VERTEX_POINT ( 'NONE', #4576 ) ;
#4470=DIRECTION ( 'NONE',  ( 1.000000000000000000, 0.000000000000000000, 0.000000000000000000 ) ) ;
#4487=ADVANCED_FACE ( 'NONE', ( #4745 ), #6488, .F. ) ;
#4498=DIRECTION ( 'NONE',  ( 0.000000000000000000, 1.000000000000000000, 0.000000000000000000 ) ) ;
#4515=DIRECTION ( 'NONE',  ( 0.000000000000000000, 0.000000000000000000, 1.000000000000000000 ) ) ;
#4516=ORIENTED_EDGE ( 'NONE', *, *, #5254, .F. ) ;
#4538=CARTESIAN_POINT ( 'NONE',  ( -99.99999999999998579, 15.67949192431120053, 0.000000000000000000 ) ) ;
#4539=VERTEX_POINT ( 'NONE', #8260 ) ;
#4540=CARTESIAN_POINT ( 'NONE',  ( -49.99999999999998579, -8.000000000000000000, 3.000000000000000000 ) ) ;
#4544=CARTESIAN_POINT ( 'NONE',  ( -120.0000000000000000, -15.00000000000001421, 83.15773105863907233 ) ) ;
#4555=ADVANCED_FACE ( 'NONE', ( #8303 ), #5693, .F. ) ;
#4576=CARTESIAN_POINT ( 'NONE',  ( -109.9999999999999289, 33.00000000000000711, 0.000000000000000000 ) ) ;
#4577=ORIENTED_EDGE ( 'NONE', *, *, #826, .F. ) ;
#4579=FACE_OUTER_BOUND ( 'NONE', #3924, .T. ) ;
#4585=VERTEX_POINT ( 'NONE', #6747 ) ;
#4593=ORIENTED_EDGE ( 'NONE', *, *, #5320, .F. ) ;
#4596=LINE ( 'NONE', #8000, #856 ) ;
#4605=VECTOR ( 'NONE', #10887, 1000.000000000000000 ) ;
#4606=DIRECTION ( 'NONE',  ( -0.000000000000000000, -0.000000000000000000, -1.000000000000000000 ) ) ;
#4618=VERTEX_POINT ( 'NONE', #3297 ) ;
#4621=DIRECTION ( 'NONE',  ( 0.000000000000000000, 0.000000000000000000, -1.000000000000000000 ) ) ;
#4626=VERTEX_POINT ( 'NONE', #8461 ) ;
#4646=ORIENTED_EDGE ( 'NONE', *, *, #2587, .T. ) ;
#4654=DIRECTION ( 'NONE',  ( 0.000000000000000000, -1.000000000000000000, 0.000000000000000000 ) ) ;
#4665=DIRECTION ( 'NONE',  ( -0.000000000000000000, 1.000000000000000000, 0.000000000000000000 ) ) ;
#4707=EDGE_CURVE ( 'NONE', #3104, #1612, #1963, .T. ) ;
#4709=DIRECTION ( 'NONE',  ( -0.000000000000000000, -1.000000000000000000, -0.000000000000000000 ) ) ;
#4714=FACE_OUTER_BOUND ( 'NONE', #115, .T. ) ;
#4730=LINE ( 'NONE', #528, #1563 ) ;
#4732=EDGE_CURVE ( 'NONE', #8685, #3802, #7799, .T. ) ;
#4736=PLANE ( 'NONE',  #1314 ) ;
#4737=ORIENTED_EDGE ( 'NONE', *, *, #10261, .T. ) ;
#4740=VERTEX_POINT ( 'NONE', #1852 ) ;
#4745=FACE_OUTER_BOUND ( 'NONE', #877, .T. ) ;
#4752=VECTOR ( 'NONE', #10055, 1000.000000000000000 ) ;
#4760=VECTOR ( 'NONE', #1490, 1000.000000000000000 ) ;
#4767=ORIENTED_EDGE ( 'NONE', *, *, #960, .F. ) ;
#4768=DIRECTION ( 'NONE',  ( 0.000000000000000000, 0.000000000000000000, -1.000000000000000000 ) ) ;
#4780=DIRECTION ( 'NONE',  ( -1.000000000000000000, -0.000000000000000000, -0.000000000000000000 ) ) ;
#4815=VECTOR ( 'NONE', #2091, 1000.000000000000000 ) ;
#4819=EDGE_LOOP ( 'NONE', ( #134, #99 ) ) ;
#4827=CIRCLE ( 'NONE', #7500, 1.099999999999989875 ) ;
#4857=CIRCLE ( 'NONE', #10720, 1.099999999999989875 ) ;
#4866=DIRECTION ( 'NONE',  ( -0.000000000000000000, -0.000000000000000000, -1.000000000000000000 ) ) ;
#4870=CARTESIAN_POINT ( 'NONE',  ( -49.99999999999998579, -15.00000000000001243, 0.000000000000000000 ) ) ;
#4875=DIRECTION ( 'NONE',  ( -1.000000000000000000, 0.000000000000000000, 0.000000000000000000 ) ) ;
#4907=CARTESIAN_POINT ( 'NONE',  ( -57.99999999999998579, -14.00000000000001243, 3.141811147483251965 ) ) ;
#4920=CARTESIAN_POINT ( 'NONE',  ( -120.0000000000000000, 3.999999999999980904, -2.000000000000000000 ) ) ;
#4923=ADVANCED_FACE ( 'NONE', ( #5835 ), #8346, .F. ) ;
#4929=DIRECTION ( 'NONE',  ( -1.000000000000000000, -3.965082230804130220E-16, 0.000000000000000000 ) ) ;
#4932=VECTOR ( 'NONE', #1286, 1000.000000000000000 ) ;
#4937=VECTOR ( 'NONE', #761, 1000.000000000000000 ) ;
#4938=VERTEX_POINT ( 'NONE', #4160 ) ;
#4948=( GEOMETRIC_REPRESENTATION_CONTEXT ( 3 ) GLOBAL_UNCERTAINTY_ASSIGNED_CONTEXT ( ( #8082 ) ) GLOBAL_UNIT_ASSIGNED_CONTEXT ( ( #7930, #7704, #256 ) ) REPRESENTATION_CONTEXT ( 'NONE', 'WORKASPACE' ) );
#4949=DIRECTION ( 'NONE',  ( 0.000000000000000000, 1.000000000000000000, -0.000000000000000000 ) ) ;
#4962=VERTEX_POINT ( 'NONE', #5780 ) ;
#4967=CARTESIAN_POINT ( 'NONE',  ( -105.0000000000000000, 2.500000000000000000, 4.000000000000000000 ) ) ;
#4974=PLANE ( 'NONE',  #346 ) ;
#4983=CARTESIAN_POINT ( 'NONE',  ( -114.9999999999999147, -43.00000000000000000, -2.000000000000000000 ) ) ;
#4993=CARTESIAN_POINT ( 'NONE',  ( -114.9999999999999289, -7.999999999999998224, -2.000000000000000000 ) ) ;
#4995=AXIS2_PLACEMENT_3D ( 'NONE', #2109, #7890, #8002 ) ;
#5003=ORIENTED_EDGE ( 'NONE', *, *, #7226, .T. ) ;
#5007=EDGE_CURVE ( 'NONE', #4740, #8859, #6523, .T. ) ;
#5057=CARTESIAN_POINT ( 'NONE',  ( -61.99999999999998579, 14.99999999999998579, 1.500000000000002220 ) ) ;
#5058=EDGE_CURVE ( 'NONE', #7983, #2258, #5151, .T. ) ;
#5068=EDGE_LOOP ( 'NONE', ( #10141, #3484, #5649, #7977 ) ) ;
#5073=DIRECTION ( 'NONE',  ( -1.000000000000000000, -2.478176394252581696E-17, 0.000000000000000000 ) ) ;
#5092=ORIENTED_EDGE ( 'NONE', *, *, #985, .F. ) ;
#5103=AXIS2_PLACEMENT_3D ( 'NONE', #6155, #9540, #1934 ) ;
#5105=ORIENTED_EDGE ( 'NONE', *, *, #5807, .T. ) ;
#5107=CARTESIAN_POINT ( 'NONE',  ( -105.0000000000000000, -2.500000000000000000, 4.000000000000000000 ) ) ;
#5120=DIRECTION ( 'NONE',  ( -2.478176394252581696E-17, 1.000000000000000000, 0.000000000000000000 ) ) ;
#5121=EDGE_CURVE ( 'NONE', #1296, #4198, #8555, .T. ) ;
#5126=ORIENTED_EDGE ( 'NONE', *, *, #6868, .F. ) ;
#5129=( NAMED_UNIT ( * ) PLANE_ANGLE_UNIT ( ) SI_UNIT ( $, .RADIAN. ) );
#5138=ADVANCED_FACE ( 'NONE', ( #7836 ), #7781, .F. ) ;
#5151=LINE ( 'NONE', #1, #9368 ) ;
#5155=LINE ( 'NONE', #10212, #9041 ) ;
#5160=CARTESIAN_POINT ( 'NONE',  ( -114.9999999999999289, -8.000000000000000000, 3.000000000000000000 ) ) ;
#5193=CARTESIAN_POINT ( 'NONE',  ( 0.000000000000000000, 0.000000000000000000, 0.000000000000000000 ) ) ;
#5198=EDGE_CURVE ( 'NONE', #3585, #4054, #10207, .T. ) ;
#5200=CARTESIAN_POINT ( 'NONE',  ( -104.9999999999999289, -7.999999999999994671, 0.000000000000000000 ) ) ;
#5203=DIRECTION ( 'NONE',  ( -1.000000000000000000, 0.000000000000000000, 0.000000000000000000 ) ) ;
#5204=EDGE_LOOP ( 'NONE', ( #3100, #448, #10962, #10666 ) ) ;
#5208=DIRECTION ( 'NONE',  ( -0.000000000000000000, -0.000000000000000000, -1.000000000000000000 ) ) ;
#5212=CARTESIAN_POINT ( 'NONE',  ( -120.0000000000000000, -4.000000000000019540, -2.000000000000000000 ) ) ;
#5229=EDGE_CURVE ( 'NONE', #4626, #4740, #2726, .T. ) ;
#5237=PLANE ( 'NONE',  #5549 ) ;
#5243=CARTESIAN_POINT ( 'NONE',  ( -76.89999999999999147, -11.50000000000000711, -2.000000000000000000 ) ) ;
#5247=VERTEX_POINT ( 'NONE', #6165 ) ;
#5254=EDGE_CURVE ( 'NONE', #6924, #7749, #8010, .T. ) ;
#5255=VECTOR ( 'NONE', #5418, 1000.000000000000000 ) ;
#5257=FACE_OUTER_BOUND ( 'NONE', #5204, .T. ) ;
#5260=CARTESIAN_POINT ( 'NONE',  ( -105.0000000000000000, -2.500000000000000000, 4.000000000000000000 ) ) ;
#5261=CARTESIAN_POINT ( 'NONE',  ( -104.9999999999999289, -16.54248688935409106, -2.000000000000000000 ) ) ;
#5287=AXIS2_PLACEMENT_3D ( 'NONE', #5352, #4470, #7817 ) ;
#5298=ORIENTED_EDGE ( 'NONE', *, *, #657, .F. ) ;
#5300=DIRECTION ( 'NONE',  ( -0.000000000000000000, -0.000000000000000000, -1.000000000000000000 ) ) ;
#5302=VECTOR ( 'NONE', #10735, 1000.000000000000000 ) ;
#5310=PLANE ( 'NONE',  #6957 ) ;
#5316=LINE ( 'NONE', #10437, #6895 ) ;
#5317=CARTESIAN_POINT ( 'NONE',  ( -120.0000000000000000, -15.00000000000001421, 5.000000000000004441 ) ) ;
#5320=EDGE_CURVE ( 'NONE', #6146, #6924, #6339, .T. ) ;
#5324=CARTESIAN_POINT ( 'NONE',  ( -77.99999999999998579, 11.49999999999999645, -2.000000000000001332 ) ) ;
#5325=ORIENTED_EDGE ( 'NONE', *, *, #10878, .F. ) ;
#5341=ORIENTED_EDGE ( 'NONE', *, *, #10184, .T. ) ;
#5342=ADVANCED_FACE ( 'NONE', ( #2897 ), #5433, .T. ) ;
#5352=CARTESIAN_POINT ( 'NONE',  ( -105.0000000000000000, -2.500000000000000000, 4.000000000000000000 ) ) ;
#5361=VECTOR ( 'NONE', #8154, 1000.000000000000000 ) ;
#5363=ORIENTED_EDGE ( 'NONE', *, *, #5229, .T. ) ;
#5378=DIRECTION ( 'NONE',  ( 0.000000000000000000, 0.000000000000000000, -1.000000000000000000 ) ) ;
#5389=DIRECTION ( 'NONE',  ( -1.000000000000000000, 0.000000000000000000, -0.000000000000000000 ) ) ;
#5403=EDGE_CURVE ( 'NONE', #2273, #2258, #5316, .T. ) ;
#5418=DIRECTION ( 'NONE',  ( 0.000000000000000000, -1.000000000000000000, 0.000000000000000000 ) ) ;
#5433=PLANE ( 'NONE',  #3696 ) ;
#5435=DIRECTION ( 'NONE',  ( -0.000000000000000000, -0.000000000000000000, -1.000000000000000000 ) ) ;
#5439=LINE ( 'NONE', #9559, #9556 ) ;
#5443=DIRECTION ( 'NONE',  ( -0.000000000000000000, -0.000000000000000000, -1.000000000000000000 ) ) ;
#5445=FACE_OUTER_BOUND ( 'NONE', #9968, .T. ) ;
#5451=CARTESIAN_POINT ( 'NONE',  ( -120.0000000000000000, -8.000000000000000000, 0.000000000000000000 ) ) ;
#5474=VECTOR ( 'NONE', #1652, 1000.000000000000000 ) ;
#5475=CARTESIAN_POINT ( 'NONE',  ( -49.99999999999998579, -15.00000000000001243, 0.000000000000000000 ) ) ;
#5490=ORIENTED_EDGE ( 'NONE', *, *, #1134, .F. ) ;
#5497=CARTESIAN_POINT ( 'NONE',  ( -120.0000000000000000, -15.00000000000001421, 0.000000000000000000 ) ) ;
#5508=EDGE_LOOP ( 'NONE', ( #1362, #4006, #46, #8485 ) ) ;
#5520=VERTEX_POINT ( 'NONE', #9003 ) ;
#5529=EDGE_CURVE ( 'NONE', #3964, #40, #2379, .T. ) ;
#5533=ORIENTED_EDGE ( 'NONE', *, *, #1100, .F. ) ;
#5539=VECTOR ( 'NONE', #6221, 1000.000000000000000 ) ;
#5549=AXIS2_PLACEMENT_3D ( 'NONE', #6318, #1080, #6085 ) ;
#5550=ADVANCED_FACE ( 'NONE', ( #3998 ), #8278, .T. ) ;
#5555=APPLICATION_CONTEXT ( 'automotive_design' ) ;
#5566=DIRECTION ( 'NONE',  ( -1.000000000000000000, 0.000000000000000000, 0.000000000000000000 ) ) ;
#5567=AXIS2_PLACEMENT_3D ( 'NONE', #6284, #5378, #1165 ) ;
#5576=EDGE_CURVE ( 'NONE', #9306, #5247, #9546, .T. ) ;
#5581=FACE_BOUND ( 'NONE', #10814, .T. ) ;
#5591=EDGE_CURVE ( 'NONE', #4539, #1599, #1469, .T. ) ;
#5602=DIRECTION ( 'NONE',  ( 0.000000000000000000, -1.000000000000000000, 0.000000000000000000 ) ) ;
#5607=FACE_OUTER_BOUND ( 'NONE', #9470, .T. ) ;
#5611=CARTESIAN_POINT ( 'NONE',  ( -120.0000000000000000, -8.000000000000000000, 3.000000000000000000 ) ) ;
#5618=VERTEX_POINT ( 'NONE', #10014 ) ;
#5629=CARTESIAN_POINT ( 'NONE',  ( -57.99999999999998579, -14.00000000000001243, -0.1418111474832477736 ) ) ;
#5649=ORIENTED_EDGE ( 'NONE', *, *, #5787, .T. ) ;
#5656=AXIS2_PLACEMENT_3D ( 'NONE', #9804, #7359, #10846 ) ;
#5665=VECTOR ( 'NONE', #5300, 1000.000000000000000 ) ;
#5672=CARTESIAN_POINT ( 'NONE',  ( -120.0000000000000000, -15.00000000000001421, 3.000000000000002665 ) ) ;
#5677=ADVANCED_FACE ( 'NONE', ( #2347 ), #3969, .F. ) ;
#5688=VERTEX_POINT ( 'NONE', #1566 ) ;
#5693=PLANE ( 'NONE',  #7865 ) ;
#5706=ORIENTED_EDGE ( 'NONE', *, *, #6586, .F. ) ;
#5714=DIRECTION ( 'NONE',  ( -1.000000000000000000, 0.000000000000000000, 0.000000000000000000 ) ) ;
#5724=ADVANCED_FACE ( 'NONE', ( #10691 ), #3081, .T. ) ;
#5726=PLANE ( 'NONE',  #914 ) ;
#5728=CARTESIAN_POINT ( 'NONE',  ( -104.9999999999999289, -15.00000000000001421, 83.15773105863907233 ) ) ;
#5753=ADVANCED_BREP_SHAPE_REPRESENTATION ( '', ( #8521, #2307 ), #4948 ) ;
#5754=EDGE_CURVE ( 'NONE', #8509, #4585, #888, .T. ) ;
#5760=DIRECTION ( 'NONE',  ( -0.000000000000000000, 1.000000000000000000, 0.000000000000000000 ) ) ;
#5766=DIRECTION ( 'NONE',  ( 1.110223024625156343E-15, 1.000000000000000000, 0.000000000000000000 ) ) ;
#5780=CARTESIAN_POINT ( 'NONE',  ( -120.0000000000000000, -8.000000000000000000, 5.000000000000004441 ) ) ;
#5781=CARTESIAN_POINT ( 'NONE',  ( 0.000000000000000000, 0.000000000000000000, -2.000000000000000000 ) ) ;
#5785=PRODUCT_CONTEXT ( 'NONE', #5555, 'mechanical' ) ;
#5787=EDGE_CURVE ( 'NONE', #9306, #1698, #111, .T. ) ;
#5791=DIRECTION ( 'NONE',  ( 1.000000000000000000, 0.000000000000000000, 0.000000000000000000 ) ) ;
#5792=CYLINDRICAL_SURFACE ( 'NONE', #3783, 1.000000000000000888 ) ;
#5807=EDGE_CURVE ( 'NONE', #6146, #4962, #9389, .T. ) ;
#5819=ORIENTED_EDGE ( 'NONE', *, *, #3167, .T. ) ;
#5827=ORIENTED_EDGE ( 'NONE', *, *, #4446, .T. ) ;
#5829=VECTOR ( 'NONE', #3527, 1000.000000000000000 ) ;
#5835=FACE_OUTER_BOUND ( 'NONE', #2054, .T. ) ;
#5843=CARTESIAN_POINT ( 'NONE',  ( -57.99999999999998579, -10.00000000000000888, 3.141811147483251965 ) ) ;
#5856=AXIS2_PLACEMENT_3D ( 'NONE', #9545, #3775, #7223 ) ;
#5868=DIRECTION ( 'NONE',  ( 0.000000000000000000, 0.000000000000000000, 1.000000000000000000 ) ) ;
#5871=ORIENTED_EDGE ( 'NONE', *, *, #10620, .T. ) ;
#5881=VECTOR ( 'NONE', #2510, 1000.000000000000000 ) ;
#5890=CARTESIAN_POINT ( 'NONE',  ( -49.99999999999998579, -4.000000000000019540, 0.000000000000000000 ) ) ;
#5893=AXIS2_PLACEMENT_3D ( 'NONE', #6598, #8307, #1481 ) ;
#5900=VERTEX_POINT ( 'NONE', #8506 ) ;
#5915=DIRECTION ( 'NONE',  ( 0.000000000000000000, 0.000000000000000000, -1.000000000000000000 ) ) ;
#5921=FACE_OUTER_BOUND ( 'NONE', #5508, .T. ) ;
#5925=EDGE_CURVE ( 'NONE', #3366, #41, #5439, .T. ) ;
#5927=EDGE_LOOP ( 'NONE', ( #2774, #9168 ) ) ;
#5958=ORIENTED_EDGE ( 'NONE', *, *, #6504, .T. ) ;
#5963=ADVANCED_FACE ( 'NONE', ( #6951 ), #3788, .F. ) ;
#5979=ORIENTED_EDGE ( 'NONE', *, *, #4707, .T. ) ;
#5986=CARTESIAN_POINT ( 'NONE',  ( -79.09999999999999432, 11.49999999999999645, 4.999999999999999112 ) ) ;
#5995=CARTESIAN_POINT ( 'NONE',  ( -114.9999999999999289, -15.00000000000001421, 5.000000000000004441 ) ) ;
#5999=CARTESIAN_POINT ( 'NONE',  ( -104.9999999999999289, -16.54248688935409106, 0.000000000000000000 ) ) ;
#6002=VECTOR ( 'NONE', #2782, 1000.000000000000000 ) ;
#6005=DIRECTION ( 'NONE',  ( -0.000000000000000000, 1.000000000000000000, 0.000000000000000000 ) ) ;
#6007=VECTOR ( 'NONE', #3443, 1000.000000000000000 ) ;
#6008=ADVANCED_FACE ( 'NONE', ( #8732, #995 ), #2904, .T. ) ;
#6014=ORIENTED_EDGE ( 'NONE', *, *, #2042, .F. ) ;
#6020=LINE ( 'NONE', #187, #10533 ) ;
#6023=EDGE_CURVE ( 'NONE', #4618, #5618, #3729, .T. ) ;
#6025=CARTESIAN_POINT ( 'NONE',  ( -49.99999999999998579, -15.00000000000001243, 3.000000000000002665 ) ) ;
#6030=DIRECTION ( 'NONE',  ( -1.000000000000000000, -2.478176394252581696E-17, 0.000000000000000000 ) ) ;
#6040=ORIENTED_EDGE ( 'NONE', *, *, #7388, .F. ) ;
#6047=ORIENTED_EDGE ( 'NONE', *, *, #7371, .F. ) ;
#6056=DIRECTION ( 'NONE',  ( 0.000000000000000000, 0.000000000000000000, -1.000000000000000000 ) ) ;
#6059=AXIS2_PLACEMENT_3D ( 'NONE', #171, #3667, #460 ) ;
#6065=CIRCLE ( 'NONE', #4995, 40.00000000000000711 ) ;
#6077=CIRCLE ( 'NONE', #425, 1.000000000000000888 ) ;
#6083=AXIS2_PLACEMENT_3D ( 'NONE', #4337, #7026, #6190 ) ;
#6085=DIRECTION ( 'NONE',  ( 0.000000000000000000, -0.000000000000000000, 1.000000000000000000 ) ) ;
#6105=ORIENTED_EDGE ( 'NONE', *, *, #9859, .T. ) ;
#6108=DIRECTION ( 'NONE',  ( -1.000000000000000000, 0.000000000000000000, 0.000000000000000000 ) ) ;
#6114=DIRECTION ( 'NONE',  ( 0.000000000000000000, -1.000000000000000000, 0.000000000000000000 ) ) ;
#6143=( NAMED_UNIT ( * ) SI_UNIT ( $, .STERADIAN. ) SOLID_ANGLE_UNIT ( ) );
#6144=LINE ( 'NONE', #10536, #9930 ) ;
#6146=VERTEX_POINT ( 'NONE', #5611 ) ;
#6147=DIRECTION ( 'NONE',  ( -0.000000000000000000, 1.000000000000000000, -0.000000000000000000 ) ) ;
#6155=CARTESIAN_POINT ( 'NONE',  ( -120.0000000000000000, -15.00000000000001421, 83.15773105863907233 ) ) ;
#6165=CARTESIAN_POINT ( 'NONE',  ( -76.89999999999997726, -11.50000000000000711, 4.999999999999999112 ) ) ;
#6175=ORIENTED_EDGE ( 'NONE', *, *, #6879, .T. ) ;
#6180=AXIS2_PLACEMENT_3D ( 'NONE', #4993, #673, #8397 ) ;
#6190=DIRECTION ( 'NONE',  ( -1.000000000000000000, 0.000000000000000000, -0.000000000000000000 ) ) ;
#6193=VECTOR ( 'NONE', #4654, 1000.000000000000000 ) ;
#6199=CARTESIAN_POINT ( 'NONE',  ( -49.99999999999998579, -2.500000000000000000, 4.000000000000000000 ) ) ;
#6200=VECTOR ( 'NONE', #5791, 1000.000000000000000 ) ;
#6203=SURFACE_SIDE_STYLE ('',( #10299 ) ) ;
#6206=( GEOMETRIC_REPRESENTATION_CONTEXT ( 3 ) GLOBAL_UNCERTAINTY_ASSIGNED_CONTEXT ( ( #3847 ) ) GLOBAL_UNIT_ASSIGNED_CONTEXT ( ( #4408, #5129, #6143 ) ) REPRESENTATION_CONTEXT ( 'NONE', 'WORKASPACE' ) );
#6221=DIRECTION ( 'NONE',  ( 1.000000000000000000, 0.000000000000000000, 0.000000000000000000 ) ) ;
#6230=EDGE_CURVE ( 'NONE', #7385, #3973, #7329, .T. ) ;
#6235=ADVANCED_FACE ( 'NONE', ( #8223 ), #611, .F. ) ;
#6237=ORIENTED_EDGE ( 'NONE', *, *, #5121, .F. ) ;
#6244=ORIENTED_EDGE ( 'NONE', *, *, #6230, .F. ) ;
#6251=CARTESIAN_POINT ( 'NONE',  ( -76.89999999999997726, 11.49999999999999645, 4.999999999999999112 ) ) ;
#6259=LINE ( 'NONE', #7260, #5361 ) ;
#6274=EDGE_CURVE ( 'NONE', #1452, #1599, #917, .T. ) ;
#6277=FACE_OUTER_BOUND ( 'NONE', #10236, .T. ) ;
#6278=EDGE_LOOP ( 'NONE', ( #7027, #3515, #306, #6377 ) ) ;
#6279=CARTESIAN_POINT ( 'NONE',  ( -61.99999999999998579, 8.000000000000000000, 1.500000000000002220 ) ) ;
#6284=CARTESIAN_POINT ( 'NONE',  ( 0.000000000000000000, 0.000000000000000000, 3.000000000000000000 ) ) ;
#6290=CARTESIAN_POINT ( 'NONE',  ( -49.99999999999998579, 3.999999999999980904, -2.000000000000000000 ) ) ;
#6318=CARTESIAN_POINT ( 'NONE',  ( -49.99998799999998766, -14.00000000000001243, 0.000000000000000000 ) ) ;
#6321=LINE ( 'NONE', #2988, #7268 ) ;
#6328=( LENGTH_UNIT ( ) NAMED_UNIT ( * ) SI_UNIT ( .MILLI., .METRE. ) );
#6335=FACE_OUTER_BOUND ( 'NONE', #6278, .T. ) ;
#6336=VERTEX_POINT ( 'NONE', #10192 ) ;
#6339=LINE ( 'NONE', #8071, #8856 ) ;
#6368=CIRCLE ( 'NONE', #1029, 1.100000000000003642 ) ;
#6375=VECTOR ( 'NONE', #5208, 1000.000000000000000 ) ;
#6377=ORIENTED_EDGE ( 'NONE', *, *, #7333, .F. ) ;
#6384=AXIS2_PLACEMENT_3D ( 'NONE', #2248, #10898, #1622 ) ;
#6412=EDGE_CURVE ( 'NONE', #2204, #8551, #9208, .T. ) ;
#6413=ORIENTED_EDGE ( 'NONE', *, *, #3617, .T. ) ;
#6418=ORIENTED_EDGE ( 'NONE', *, *, #10500, .F. ) ;
#6423=ADVANCED_FACE ( 'NONE', ( #6870 ), #4974, .F. ) ;
#6446=VECTOR ( 'NONE', #4709, 1000.000000000000000 ) ;
#6450=DIRECTION ( 'NONE',  ( 1.000000000000000000, 0.000000000000000000, 0.000000000000000000 ) ) ;
#6459=FACE_BOUND ( 'NONE', #4819, .T. ) ;
#6461=AXIS2_PLACEMENT_3D ( 'NONE', #7237, #4621, #8020 ) ;
#6467=CARTESIAN_POINT ( 'NONE',  ( -149.9999999999999716, -8.000000000000000000, 0.000000000000000000 ) ) ;
#6476=CARTESIAN_POINT ( 'NONE',  ( -77.99999999999998579, -11.50000000000000711, -2.000000000000000000 ) ) ;
#6488=PLANE ( 'NONE',  #1650 ) ;
#6489=EDGE_LOOP ( 'NONE', ( #10909, #5105, #6902, #159, #9012, #6649, #7489, #7800, #10753, #7884 ) ) ;
#6504=EDGE_CURVE ( 'NONE', #7831, #1714, #2705, .T. ) ;
#6506=CYLINDRICAL_SURFACE ( 'NONE', #10516, 40.00000000000000711 ) ;
#6516=CARTESIAN_POINT ( 'NONE',  ( -114.9999999999999289, -15.00000000000001421, -2.000000000000000000 ) ) ;
#6523=LINE ( 'NONE', #1410, #7071 ) ;
#6532=DIRECTION ( 'NONE',  ( 0.000000000000000000, 0.000000000000000000, 1.000000000000000000 ) ) ;
#6534=CARTESIAN_POINT ( 'NONE',  ( -105.0000000000000000, -2.500000000000000000, 4.000000000000000000 ) ) ;
#6538=STYLED_ITEM('',(#11013),#8521);
#6545=EDGE_CURVE ( 'NONE', #5247, #2376, #1872, .T. ) ;
#6550=ORIENTED_EDGE ( 'NONE', *, *, #9999, .F. ) ;
#6560=VECTOR ( 'NONE', #1053, 1000.000000000000000 ) ;
#6563=FACE_OUTER_BOUND ( 'NONE', #7314, .T. ) ;
#6571=COLOUR_RGB ( '',0.8941176470588234615, 0.8941176470588234615, 0.8941176470588234615 ) ;
#6574=DIRECTION ( 'NONE',  ( 1.000000000000000000, 0.000000000000000000, 0.000000000000000000 ) ) ;
#6576=ORIENTED_EDGE ( 'NONE', *, *, #7371, .T. ) ;
#6577=LINE ( 'NONE', #5728, #214 ) ;
#6586=EDGE_CURVE ( 'NONE', #4618, #7831, #3531, .T. ) ;
#6590=ORIENTED_EDGE ( 'NONE', *, *, #3617, .F. ) ;
#6596=ORIENTED_EDGE ( 'NONE', *, *, #9267, .F. ) ;
#6598=CARTESIAN_POINT ( 'NONE',  ( -104.9999999999999289, -7.999999999999994671, -2.000000000000000000 ) ) ;
#6602=EDGE_CURVE ( 'NONE', #4626, #6858, #201, .T. ) ;
#6605=LINE ( 'NONE', #6702, #10232 ) ;
#6606=ORIENTED_EDGE ( 'NONE', *, *, #6658, .T. ) ;
#6608=LINE ( 'NONE', #8112, #4760 ) ;
#6623=ORIENTED_EDGE ( 'NONE', *, *, #657, .T. ) ;
#6624=CARTESIAN_POINT ( 'NONE',  ( -49.99999999999998579, -4.000000000000019540, -2.000000000000000000 ) ) ;
#6627=VECTOR ( 'NONE', #2341, 1000.000000000000000 ) ;
#6639=CARTESIAN_POINT ( 'NONE',  ( -49.99999999999998579, -15.00000000000001243, -2.000000000000000000 ) ) ;
#6640=ORIENTED_EDGE ( 'NONE', *, *, #5320, .T. ) ;
#6649=ORIENTED_EDGE ( 'NONE', *, *, #2411, .T. ) ;
#6658=EDGE_CURVE ( 'NONE', #1296, #3152, #7992, .T. ) ;
#6674=ORIENTED_EDGE ( 'NONE', *, *, #6602, .F. ) ;
#6679=DIRECTION ( 'NONE',  ( -1.000000000000000000, 0.000000000000000000, 0.000000000000000000 ) ) ;
#6685=LINE ( 'NONE', #2452, #5881 ) ;
#6689=DIRECTION ( 'NONE',  ( -0.000000000000000000, 1.000000000000000000, -0.000000000000000000 ) ) ;
#6702=CARTESIAN_POINT ( 'NONE',  ( -120.0000000000000000, 3.999999999999980904, -2.000000000000000000 ) ) ;
#6704=EDGE_CURVE ( 'NONE', #4361, #2204, #536, .T. ) ;
#6739=ORIENTED_EDGE ( 'NONE', *, *, #7073, .T. ) ;
#6747=CARTESIAN_POINT ( 'NONE',  ( -120.0000000000000000, 14.99999999999998579, 0.000000000000000000 ) ) ;
#6768=ORIENTED_EDGE ( 'NONE', *, *, #6023, .F. ) ;
#6772=ORIENTED_EDGE ( 'NONE', *, *, #1644, .T. ) ;
#6780=LINE ( 'NONE', #4155, #7811 ) ;
#6785=DIRECTION ( 'NONE',  ( -0.000000000000000000, 1.000000000000000000, -0.000000000000000000 ) ) ;
#6796=DIRECTION ( 'NONE',  ( -0.000000000000000000, -0.000000000000000000, -1.000000000000000000 ) ) ;
#6803=DIRECTION ( 'NONE',  ( -1.000000000000000000, -0.000000000000000000, -0.000000000000000000 ) ) ;
#6804=ORIENTED_EDGE ( 'NONE', *, *, #1694, .T. ) ;
#6809=PLANE ( 'NONE',  #6083 ) ;
#6813=AXIS2_PLACEMENT_3D ( 'NONE', #4544, #8784, #7950 ) ;
#6816=DIRECTION ( 'NONE',  ( -2.478176394252581696E-17, 1.000000000000000000, 0.000000000000000000 ) ) ;
#6829=EDGE_CURVE ( 'NONE', #3291, #1599, #2305, .T. ) ;
#6841=DIRECTION ( 'NONE',  ( -0.000000000000000000, -0.000000000000000000, -1.000000000000000000 ) ) ;
#6846=LINE ( 'NONE', #10168, #10812 ) ;
#6857=LINE ( 'NONE', #4393, #3795 ) ;
#6858=VERTEX_POINT ( 'NONE', #892 ) ;
#6868=EDGE_CURVE ( 'NONE', #6924, #4054, #4380, .T. ) ;
#6870=FACE_OUTER_BOUND ( 'NONE', #9774, .T. ) ;
#6879=EDGE_CURVE ( 'NONE', #8912, #211, #9449, .T. ) ;
#6891=LINE ( 'NONE', #1888, #9460 ) ;
#6895=VECTOR ( 'NONE', #2061, 1000.000000000000000 ) ;
#6900=VECTOR ( 'NONE', #9444, 1000.000000000000000 ) ;
#6902=ORIENTED_EDGE ( 'NONE', *, *, #6974, .T. ) ;
#6924=VERTEX_POINT ( 'NONE', #5160 ) ;
#6932=DIRECTION ( 'NONE',  ( -1.000000000000000000, 0.000000000000000000, 0.000000000000000000 ) ) ;
#6933=DIRECTION ( 'NONE',  ( 0.000000000000000000, 0.000000000000000000, 1.000000000000000000 ) ) ;
#6937=DIRECTION ( 'NONE',  ( -1.000000000000000000, -0.000000000000000000, -0.000000000000000000 ) ) ;
#6950=CARTESIAN_POINT ( 'NONE',  ( -109.9999999999999289, 33.00000000000000711, -2.000000000000000000 ) ) ;
#6951=FACE_OUTER_BOUND ( 'NONE', #8983, .T. ) ;
#6955=DIRECTION ( 'NONE',  ( -0.000000000000000000, -0.000000000000000000, 1.000000000000000000 ) ) ;
#6957=AXIS2_PLACEMENT_3D ( 'NONE', #9602, #7942, #1995 ) ;
#6962=CARTESIAN_POINT ( 'NONE',  ( -105.0000000000000000, 2.500000000000000000, 4.000000000000000000 ) ) ;
#6974=EDGE_CURVE ( 'NONE', #4962, #8694, #6846, .T. ) ;
#6978=ORIENTED_EDGE ( 'NONE', *, *, #9340, .F. ) ;
#6983=LINE ( 'NONE', #7036, #5829 ) ;
#6988=DIRECTION ( 'NONE',  ( 0.000000000000000000, 0.000000000000000000, 1.000000000000000000 ) ) ;
#6991=ORIENTED_EDGE ( 'NONE', *, *, #141, .T. ) ;
#6996=CARTESIAN_POINT ( 'NONE',  ( -79.09999999999998010, 11.49999999999999645, -2.000000000000001332 ) ) ;
#6997=ORIENTED_EDGE ( 'NONE', *, *, #2100, .T. ) ;
#7009=CARTESIAN_POINT ( 'NONE',  ( -120.0000000000000000, -4.000000000000019540, -2.000000000000000000 ) ) ;
#7018=EDGE_LOOP ( 'NONE', ( #9185, #10582, #7485, #3026 ) ) ;
#7026=DIRECTION ( 'NONE',  ( 0.000000000000000000, 0.000000000000000000, -1.000000000000000000 ) ) ;
#7027=ORIENTED_EDGE ( 'NONE', *, *, #5925, .F. ) ;
#7036=CARTESIAN_POINT ( 'NONE',  ( -120.0000000000000000, 14.99999999999998579, 83.15773105863907233 ) ) ;
#7049=VERTEX_POINT ( 'NONE', #462 ) ;
#7066=DIRECTION ( 'NONE',  ( 0.000000000000000000, 0.000000000000000000, -1.000000000000000000 ) ) ;
#7071=VECTOR ( 'NONE', #9961, 1000.000000000000000 ) ;
#7073=EDGE_CURVE ( 'NONE', #5247, #9306, #9575, .T. ) ;
#7078=AXIS2_PLACEMENT_3D ( 'NONE', #1501, #512, #4100 ) ;
#7086=VECTOR ( 'NONE', #7708, 1000.000000000000000 ) ;
#7094=DIRECTION ( 'NONE',  ( 0.000000000000000000, 0.000000000000000000, -1.000000000000000000 ) ) ;
#7109=VECTOR ( 'NONE', #5602, 1000.000000000000000 ) ;
#7113=PLANE ( 'NONE',  #5856 ) ;
#7123=LINE ( 'NONE', #6290, #9745 ) ;
#7145=ORIENTED_EDGE ( 'NONE', *, *, #118, .F. ) ;
#7151=ORIENTED_EDGE ( 'NONE', *, *, #5807, .F. ) ;
#7164=AXIS2_PLACEMENT_3D ( 'NONE', #10566, #5566, #10680 ) ;
#7167=LINE ( 'NONE', #10550, #9986 ) ;
#7177=ADVANCED_FACE ( 'NONE', ( #285, #8849, #3669 ), #9679, .F. ) ;
#7182=ORIENTED_EDGE ( 'NONE', *, *, #826, .T. ) ;
#7199=ORIENTED_EDGE ( 'NONE', *, *, #6412, .F. ) ;
#7223=DIRECTION ( 'NONE',  ( 0.000000000000000000, 0.000000000000000000, -1.000000000000000000 ) ) ;
#7226=EDGE_CURVE ( 'NONE', #5688, #3585, #518, .T. ) ;
#7228=PLANE ( 'NONE',  #5567 ) ;
#7230=CARTESIAN_POINT ( 'NONE',  ( -79.09999999999999432, -11.50000000000000711, 4.999999999999999112 ) ) ;
#7237=CARTESIAN_POINT ( 'NONE',  ( -99.99999999999998579, 15.67949192431120053, -2.000000000000000000 ) ) ;
#7239=EDGE_LOOP ( 'NONE', ( #6640, #9170, #7553, #7151 ) ) ;
#7244=ORIENTED_EDGE ( 'NONE', *, *, #3607, .T. ) ;
#7252=EDGE_CURVE ( 'NONE', #9653, #9204, #2435, .T. ) ;
#7259=CIRCLE ( 'NONE', #10964, 1.000000000000000888 ) ;
#7260=CARTESIAN_POINT ( 'NONE',  ( -49.99999999999998579, -15.00000000000001243, -0.1418111474832534080 ) ) ;
#7261=ORIENTED_EDGE ( 'NONE', *, *, #10836, .T. ) ;
#7265=AXIS2_PLACEMENT_3D ( 'NONE', #7289, #1500, #566 ) ;
#7268=VECTOR ( 'NONE', #1565, 1000.000000000000000 ) ;
#7273=ORIENTED_EDGE ( 'NONE', *, *, #2042, .T. ) ;
#7289=CARTESIAN_POINT ( 'NONE',  ( -77.99999999999998579, -11.50000000000000711, 4.999999999999999112 ) ) ;
#7293=ORIENTED_EDGE ( 'NONE', *, *, #10731, .T. ) ;
#7295=EDGE_CURVE ( 'NONE', #6858, #3994, #8238, .T. ) ;
#7298=DIRECTION ( 'NONE',  ( -0.000000000000000000, -0.000000000000000000, -1.000000000000000000 ) ) ;
#7314=EDGE_LOOP ( 'NONE', ( #9312, #863, #29, #7199 ) ) ;
#7329=LINE ( 'NONE', #10820, #6193 ) ;
#7330=ORIENTED_EDGE ( 'NONE', *, *, #4707, .F. ) ;
#7333=EDGE_CURVE ( 'NONE', #41, #2258, #3954, .T. ) ;
#7335=ORIENTED_EDGE ( 'NONE', *, *, #795, .F. ) ;
#7338=DIRECTION ( 'NONE',  ( -3.965082230804130220E-16, 1.000000000000000000, -0.000000000000000000 ) ) ;
#7345=CARTESIAN_POINT ( 'NONE',  ( -109.9999999999999289, 33.00000000000000711, 0.000000000000000000 ) ) ;
#7359=DIRECTION ( 'NONE',  ( 0.000000000000000000, -0.000000000000000000, 1.000000000000000000 ) ) ;
#7371=EDGE_CURVE ( 'NONE', #40, #2188, #3070, .T. ) ;
#7372=EDGE_CURVE ( 'NONE', #3431, #4466, #571, .T. ) ;
#7380=CARTESIAN_POINT ( 'NONE',  ( -49.99999999999998579, -10.00000000000000888, 3.141811147483255073 ) ) ;
#7381=EDGE_LOOP ( 'NONE', ( #5490, #5958, #870, #6768 ) ) ;
#7385=VERTEX_POINT ( 'NONE', #3120 ) ;
#7388=EDGE_CURVE ( 'NONE', #4054, #4962, #4312, .T. ) ;
#7390=FACE_OUTER_BOUND ( 'NONE', #4180, .T. ) ;
#7394=FACE_OUTER_BOUND ( 'NONE', #3706, .T. ) ;
#7398=ORIENTED_EDGE ( 'NONE', *, *, #3167, .F. ) ;
#7419=DIRECTION ( 'NONE',  ( -1.000000000000000000, 0.000000000000000000, -0.000000000000000000 ) ) ;
#7427=AXIS2_PLACEMENT_3D ( 'NONE', #5781, #631, #1412 ) ;
#7428=ADVANCED_FACE ( 'NONE', ( #3377 ), #8493, .F. ) ;
#7456=CIRCLE ( 'NONE', #1250, 1.000000000000000888 ) ;
#7457=CARTESIAN_POINT ( 'NONE',  ( -49.99998799999998766, 0.000000000000000000, -0.1418111474832477736 ) ) ;
#7459=CARTESIAN_POINT ( 'NONE',  ( -120.0000000000000000, 15.67949192431120053, 83.15773105863907233 ) ) ;
#7460=PRODUCT_DEFINITION_FORMATION_WITH_SPECIFIED_SOURCE ( 'ANY', '', #48, .NOT_KNOWN. ) ;
#7465=CARTESIAN_POINT ( 'NONE',  ( -76.89999999999999147, 11.49999999999999645, -2.000000000000001332 ) ) ;
#7485=ORIENTED_EDGE ( 'NONE', *, *, #7867, .T. ) ;
#7489=ORIENTED_EDGE ( 'NONE', *, *, #10310, .T. ) ;
#7492=AXIS2_PLACEMENT_3D ( 'NONE', #2472, #5120, #10809 ) ;
#7494=DIRECTION ( 'NONE',  ( -1.000000000000000000, 0.000000000000000000, 0.000000000000000000 ) ) ;
#7496=CARTESIAN_POINT ( 'NONE',  ( -49.99999999999998579, 14.99999999999998579, 83.15773105863907233 ) ) ;
#7497=CARTESIAN_POINT ( 'NONE',  ( -149.9999999999999716, 8.000000000000000000, 3.000000000000000000 ) ) ;
#7500=AXIS2_PLACEMENT_3D ( 'NONE', #9070, #7298, #3073 ) ;
#7517=CARTESIAN_POINT ( 'NONE',  ( -49.99999999999998579, 14.99999999999998579, -2.000000000000000000 ) ) ;
#7525=EDGE_CURVE ( 'NONE', #8694, #3964, #6780, .T. ) ;
#7538=VERTEX_POINT ( 'NONE', #5986 ) ;
#7545=EDGE_LOOP ( 'NONE', ( #4428, #7625, #3209, #3933 ) ) ;
#7553=ORIENTED_EDGE ( 'NONE', *, *, #7388, .T. ) ;
#7566=CARTESIAN_POINT ( 'NONE',  ( -120.0000000000000000, -8.000000000000000000, -2.000000000000000000 ) ) ;
#7576=ORIENTED_EDGE ( 'NONE', *, *, #5198, .T. ) ;
#7591=AXIS2_PLACEMENT_3D ( 'NONE', #6476, #10009, #6679 ) ;
#7598=VECTOR ( 'NONE', #220, 1000.000000000000000 ) ;
#7601=ORIENTED_EDGE ( 'NONE', *, *, #1495, .F. ) ;
#7608=ORIENTED_EDGE ( 'NONE', *, *, #10027, .F. ) ;
#7625=ORIENTED_EDGE ( 'NONE', *, *, #964, .T. ) ;
#7636=VECTOR ( 'NONE', #3421, 1000.000000000000000 ) ;
#7640=ORIENTED_EDGE ( 'NONE', *, *, #7295, .T. ) ;
#7646=ADVANCED_FACE ( 'NONE', ( #6335 ), #7113, .T. ) ;
#7648=CARTESIAN_POINT ( 'NONE',  ( -109.9999999999999289, 33.00000000000000711, -2.000000000000000000 ) ) ;
#7655=VECTOR ( 'NONE', #6803, 1000.000000000000000 ) ;
#7662=CARTESIAN_POINT ( 'NONE',  ( -149.9999999999999716, -8.000000000000000000, 0.000000000000000000 ) ) ;
#7675=AXIS2_PLACEMENT_3D ( 'NONE', #330, #10554, #392 ) ;
#7704=( NAMED_UNIT ( * ) PLANE_ANGLE_UNIT ( ) SI_UNIT ( $, .RADIAN. ) );
#7707=ORIENTED_EDGE ( 'NONE', *, *, #7372, .F. ) ;
#7708=DIRECTION ( 'NONE',  ( -0.000000000000000000, 1.000000000000000000, 0.000000000000000000 ) ) ;
#7709=ORIENTED_EDGE ( 'NONE', *, *, #7864, .F. ) ;
#7727=DIRECTION ( 'NONE',  ( -1.000000000000000000, 0.000000000000000000, 0.000000000000000000 ) ) ;
#7735=ORIENTED_EDGE ( 'NONE', *, *, #2693, .F. ) ;
#7737=DIRECTION ( 'NONE',  ( 0.000000000000000000, 0.000000000000000000, 1.000000000000000000 ) ) ;
#7744=ORIENTED_EDGE ( 'NONE', *, *, #851, .T. ) ;
#7749=VERTEX_POINT ( 'NONE', #4540 ) ;
#7753=EDGE_CURVE ( 'NONE', #8685, #2572, #7456, .T. ) ;
#7774=DIRECTION ( 'NONE',  ( -1.000000000000000000, -3.469446951953572774E-16, 0.000000000000000000 ) ) ;
#7776=VECTOR ( 'NONE', #4665, 1000.000000000000000 ) ;
#7781=CYLINDRICAL_SURFACE ( 'NONE', #2283, 1.000000000000000888 ) ;
#7793=DIRECTION ( 'NONE',  ( 0.000000000000000000, 0.000000000000000000, -1.000000000000000000 ) ) ;
#7799=LINE ( 'NONE', #2571, #4454 ) ;
#7800=ORIENTED_EDGE ( 'NONE', *, *, #8536, .T. ) ;
#7806=ORIENTED_EDGE ( 'NONE', *, *, #5198, .F. ) ;
#7811=VECTOR ( 'NONE', #10317, 1000.000000000000000 ) ;
#7812=CARTESIAN_POINT ( 'NONE',  ( -105.0000000000000000, -2.500000000000000000, 3.000000000000000000 ) ) ;
#7813=ORIENTED_EDGE ( 'NONE', *, *, #4377, .T. ) ;
#7817=DIRECTION ( 'NONE',  ( 0.000000000000000000, 0.000000000000000000, -1.000000000000000000 ) ) ;
#7819=ORIENTED_EDGE ( 'NONE', *, *, #7525, .F. ) ;
#7823=ORIENTED_EDGE ( 'NONE', *, *, #1694, .F. ) ;
#7831=VERTEX_POINT ( 'NONE', #9885 ) ;
#7836=FACE_OUTER_BOUND ( 'NONE', #7381, .T. ) ;
#7845=ORIENTED_EDGE ( 'NONE', *, *, #8698, .T. ) ;
#7855=EDGE_LOOP ( 'NONE', ( #489, #726, #8999, #205 ) ) ;
#7864=EDGE_CURVE ( 'NONE', #9204, #3994, #10664, .T. ) ;
#7865=AXIS2_PLACEMENT_3D ( 'NONE', #3141, #10803, #1577 ) ;
#7867=EDGE_CURVE ( 'NONE', #2572, #570, #3157, .T. ) ;
#7884=ORIENTED_EDGE ( 'NONE', *, *, #6829, .F. ) ;
#7890=DIRECTION ( 'NONE',  ( -0.000000000000000000, -0.000000000000000000, 1.000000000000000000 ) ) ;
#7891=ORIENTED_EDGE ( 'NONE', *, *, #10878, .T. ) ;
#7930=( LENGTH_UNIT ( ) NAMED_UNIT ( * ) SI_UNIT ( .MILLI., .METRE. ) );
#7942=DIRECTION ( 'NONE',  ( 0.000000000000000000, 1.000000000000000000, 0.000000000000000000 ) ) ;
#7950=DIRECTION ( 'NONE',  ( 0.000000000000000000, 0.000000000000000000, -1.000000000000000000 ) ) ;
#7976=FACE_OUTER_BOUND ( 'NONE', #1340, .T. ) ;
#7977=ORIENTED_EDGE ( 'NONE', *, *, #2887, .T. ) ;
#7983=VERTEX_POINT ( 'NONE', #3888 ) ;
#7992=LINE ( 'NONE', #6534, #6200 ) ;
#8000=CARTESIAN_POINT ( 'NONE',  ( -49.99999999999998579, -15.00000000000001243, -2.000000000000000000 ) ) ;
#8002=DIRECTION ( 'NONE',  ( -1.000000000000000000, 0.000000000000000000, 0.000000000000000000 ) ) ;
#8003=ORIENTED_EDGE ( 'NONE', *, *, #795, .T. ) ;
#8006=ORIENTED_EDGE ( 'NONE', *, *, #2401, .T. ) ;
#8010=LINE ( 'NONE', #3660, #4932 ) ;
#8020=DIRECTION ( 'NONE',  ( -1.000000000000000000, 0.000000000000000000, 0.000000000000000000 ) ) ;
#8049=AXIS2_PLACEMENT_3D ( 'NONE', #2038, #7094, #372 ) ;
#8062=CARTESIAN_POINT ( 'NONE',  ( -77.99999999999998579, 11.49999999999999645, -2.000000000000000000 ) ) ;
#8070=CARTESIAN_POINT ( 'NONE',  ( -104.9999999999999289, -7.999999999999994671, -2.000000000000000000 ) ) ;
#8071=CARTESIAN_POINT ( 'NONE',  ( -149.9999999999999716, -8.000000000000000000, 3.000000000000000000 ) ) ;
#8072=LINE ( 'NONE', #5261, #10794 ) ;
#8078=EDGE_CURVE ( 'NONE', #8566, #41, #4193, .T. ) ;
#8082=UNCERTAINTY_MEASURE_WITH_UNIT (LENGTH_MEASURE( 1.000000000000000082E-05 ), #7930, 'distance_accuracy_value', 'NONE');
#8094=CARTESIAN_POINT ( 'NONE',  ( -57.99999999999998579, -10.00000000000001066, -0.1418111474832477736 ) ) ;
#8112=CARTESIAN_POINT ( 'NONE',  ( -79.09999999999998010, 11.49999999999999645, -2.000000000000000000 ) ) ;
#8120=CARTESIAN_POINT ( 'NONE',  ( -114.9999999999999289, -7.999999999999998224, 5.000000000000004441 ) ) ;
#8122=CARTESIAN_POINT ( 'NONE',  ( -76.89999999999999147, 11.49999999999999645, -2.000000000000000000 ) ) ;
#8128=EDGE_LOOP ( 'NONE', ( #10315, #3232 ) ) ;
#8146=DIRECTION ( 'NONE',  ( 0.000000000000000000, 0.000000000000000000, -1.000000000000000000 ) ) ;
#8154=DIRECTION ( 'NONE',  ( 0.000000000000000000, 1.000000000000000000, 0.000000000000000000 ) ) ;
#8158=ADVANCED_FACE ( 'NONE', ( #8771 ), #378, .F. ) ;
#8177=PLANE ( 'NONE',  #2210 ) ;
#8178=DIRECTION ( 'NONE',  ( -0.000000000000000000, -0.000000000000000000, -1.000000000000000000 ) ) ;
#8179=FACE_BOUND ( 'NONE', #464, .T. ) ;
#8184=ORIENTED_EDGE ( 'NONE', *, *, #3607, .F. ) ;
#8188=EDGE_LOOP ( 'NONE', ( #8006, #2036, #6772, #4250 ) ) ;
#8215=( NAMED_UNIT ( * ) PLANE_ANGLE_UNIT ( ) SI_UNIT ( $, .RADIAN. ) );
#8217=ORIENTED_EDGE ( 'NONE', *, *, #7525, .T. ) ;
#8221=CARTESIAN_POINT ( 'NONE',  ( -120.0000000000000000, 14.99999999999998579, 0.000000000000000000 ) ) ;
#8223=FACE_OUTER_BOUND ( 'NONE', #10866, .T. ) ;
#8227=AXIS2_PLACEMENT_3D ( 'NONE', #10769, #10825, #5766 ) ;
#8229=VERTEX_POINT ( 'NONE', #9594 ) ;
#8238=LINE ( 'NONE', #6467, #710 ) ;
#8241=EDGE_CURVE ( 'NONE', #2188, #3431, #8712, .T. ) ;
#8250=SHAPE_DEFINITION_REPRESENTATION ( #1831, #2047 ) ;
#8252=EDGE_CURVE ( 'NONE', #4539, #10433, #9709, .T. ) ;
#8260=CARTESIAN_POINT ( 'NONE',  ( -49.99999999999998579, 8.000000000000000000, 0.000000000000000000 ) ) ;
#8270=DIRECTION ( 'NONE',  ( -1.000000000000000000, 0.000000000000000000, 0.000000000000000000 ) ) ;
#8276=DIRECTION ( 'NONE',  ( -1.000000000000000000, 0.000000000000000000, 0.000000000000000000 ) ) ;
#8278=PLANE ( 'NONE',  #10431 ) ;
#8285=CARTESIAN_POINT ( 'NONE',  ( -57.99999999999998579, -10.00000000000001066, 5.282956808509874826E-15 ) ) ;
#8303=FACE_OUTER_BOUND ( 'NONE', #7239, .T. ) ;
#8307=DIRECTION ( 'NONE',  ( 1.000000000000000000, 3.965082230804130220E-16, -0.000000000000000000 ) ) ;
#8320=CARTESIAN_POINT ( 'NONE',  ( -61.99999999999998579, 14.99999999999998579, 2.500000000000003109 ) ) ;
#8321=VECTOR ( 'NONE', #6841, 1000.000000000000000 ) ;
#8346=PLANE ( 'NONE',  #6180 ) ;
#8348=PRODUCT_DEFINITION_CONTEXT ( 'detailed design', #10377, 'design' ) ;
#8351=LINE ( 'NONE', #4118, #862 ) ;
#8374=CARTESIAN_POINT ( 'NONE',  ( -114.9999999999999289, -7.999999999999998224, -2.000000000000000000 ) ) ;
#8384=DIRECTION ( 'NONE',  ( 3.965082230804130220E-16, -1.000000000000000000, 0.000000000000000000 ) ) ;
#8397=DIRECTION ( 'NONE',  ( -1.000000000000000000, -3.469446951953572774E-16, 0.000000000000000000 ) ) ;
#8410=DIRECTION ( 'NONE',  ( 0.000000000000000000, 0.000000000000000000, -1.000000000000000000 ) ) ;
#8425=DIRECTION ( 'NONE',  ( -1.000000000000000000, 0.000000000000000000, 0.000000000000000000 ) ) ;
#8437=DIRECTION ( 'NONE',  ( -3.965082230804130220E-16, 1.000000000000000000, -0.000000000000000000 ) ) ;
#8461=CARTESIAN_POINT ( 'NONE',  ( -114.9999999999999289, -7.999999999999998224, -2.000000000000000000 ) ) ;
#8485=ORIENTED_EDGE ( 'NONE', *, *, #9509, .T. ) ;
#8491=LINE ( 'NONE', #7662, #5539 ) ;
#8492=EDGE_LOOP ( 'NONE', ( #574, #10135, #7813, #9924 ) ) ;
#8493=CYLINDRICAL_SURFACE ( 'NONE', #8887, 1.099999999999989875 ) ;
#8498=VECTOR ( 'NONE', #6955, 1000.000000000000000 ) ;
#8506=CARTESIAN_POINT ( 'NONE',  ( -109.9999999999999289, 33.00000000000000711, -2.000000000000000000 ) ) ;
#8509=VERTEX_POINT ( 'NONE', #1380 ) ;
#8512=CARTESIAN_POINT ( 'NONE',  ( -79.09999999999998010, -11.50000000000000711, -2.000000000000001332 ) ) ;
#8513=VECTOR ( 'NONE', #7774, 1000.000000000000000 ) ;
#8521=MANIFOLD_SOLID_BREP ( 'AdvancedHole1', #2514 ) ;
#8528=CARTESIAN_POINT ( 'NONE',  ( -61.99999999999998579, 8.000000000000000000, 0.5000000000000013323 ) ) ;
#8536=EDGE_CURVE ( 'NONE', #10601, #1452, #6605, .T. ) ;
#8551=VERTEX_POINT ( 'NONE', #9149 ) ;
#8555=LINE ( 'NONE', #5260, #6375 ) ;
#8566=VERTEX_POINT ( 'NONE', #7380 ) ;
#8568=DIRECTION ( 'NONE',  ( -0.000000000000000000, 1.000000000000000000, -0.000000000000000000 ) ) ;
#8580=VECTOR ( 'NONE', #3955, 1000.000000000000000 ) ;
#8583=ORIENTED_EDGE ( 'NONE', *, *, #7295, .F. ) ;
#8586=LINE ( 'NONE', #2529, #10604 ) ;
#8589=CARTESIAN_POINT ( 'NONE',  ( -77.99999999999998579, 11.49999999999999645, -2.000000000000000000 ) ) ;
#8616=CARTESIAN_POINT ( 'NONE',  ( -49.99998799999998766, -14.00000000000001243, 3.141811147483251965 ) ) ;
#8621=CARTESIAN_POINT ( 'NONE',  ( -49.99999999999998579, -15.00000000000001243, 83.15773105863907233 ) ) ;
#8639=ORIENTED_EDGE ( 'NONE', *, *, #8252, .T. ) ;
#8646=MECHANICAL_DESIGN_GEOMETRIC_PRESENTATION_REPRESENTATION('',(#6538),#1206);
#8648=CARTESIAN_POINT ( 'NONE',  ( -61.99999999999998579, 14.99999999999998579, 1.500000000000002220 ) ) ;
#8664=CARTESIAN_POINT ( 'NONE',  ( -61.99999999999998579, 14.99999999999998579, 1.500000000000002220 ) ) ;
#8665=DIRECTION ( 'NONE',  ( -1.000000000000000000, -2.478176394252581696E-17, 0.000000000000000000 ) ) ;
#8680=VECTOR ( 'NONE', #5868, 1000.000000000000000 ) ;
#8685=VERTEX_POINT ( 'NONE', #8528 ) ;
#8694=VERTEX_POINT ( 'NONE', #4236 ) ;
#8698=EDGE_CURVE ( 'NONE', #8768, #9263, #8586, .T. ) ;
#8703=ORIENTED_EDGE ( 'NONE', *, *, #9098, .F. ) ;
#8712=LINE ( 'NONE', #1030, #9010 ) ;
#8715=ORIENTED_EDGE ( 'NONE', *, *, #9509, .F. ) ;
#8732=FACE_BOUND ( 'NONE', #8128, .T. ) ;
#8738=LINE ( 'NONE', #5107, #2707 ) ;
#8744=EDGE_CURVE ( 'NONE', #544, #7749, #2639, .T. ) ;
#8753=ORIENTED_EDGE ( 'NONE', *, *, #10813, .F. ) ;
#8768=VERTEX_POINT ( 'NONE', #2090 ) ;
#8770=DIRECTION ( 'NONE',  ( -0.000000000000000000, -0.000000000000000000, 1.000000000000000000 ) ) ;
#8771=FACE_OUTER_BOUND ( 'NONE', #7018, .T. ) ;
#8784=DIRECTION ( 'NONE',  ( 1.000000000000000000, 0.000000000000000000, 0.000000000000000000 ) ) ;
#8847=ORIENTED_EDGE ( 'NONE', *, *, #9267, .T. ) ;
#8848=ADVANCED_FACE ( 'NONE', ( #3676 ), #9743, .F. ) ;
#8849=FACE_BOUND ( 'NONE', #1977, .T. ) ;
#8851=CYLINDRICAL_SURFACE ( 'NONE', #6461, 20.00000000000000355 ) ;
#8856=VECTOR ( 'NONE', #454, 1000.000000000000000 ) ;
#8859=VERTEX_POINT ( 'NONE', #5451 ) ;
#8865=CARTESIAN_POINT ( 'NONE',  ( 0.000000000000000000, 0.000000000000000000, -2.000000000000000000 ) ) ;
#8869=ORIENTED_EDGE ( 'NONE', *, *, #5058, .T. ) ;
#8887=AXIS2_PLACEMENT_3D ( 'NONE', #9277, #2550, #5203 ) ;
#8901=LINE ( 'NONE', #5317, #2275 ) ;
#8912=VERTEX_POINT ( 'NONE', #2391 ) ;
#8924=ORIENTED_EDGE ( 'NONE', *, *, #2925, .T. ) ;
#8926=ORIENTED_EDGE ( 'NONE', *, *, #7864, .T. ) ;
#8934=CARTESIAN_POINT ( 'NONE',  ( -49.99999999999998579, -15.00000000000001243, 3.141811147483255962 ) ) ;
#8938=ORIENTED_EDGE ( 'NONE', *, *, #572, .T. ) ;
#8952=ORIENTED_EDGE ( 'NONE', *, *, #6602, .T. ) ;
#8962=ORIENTED_EDGE ( 'NONE', *, *, #6879, .F. ) ;
#8967=ADVANCED_FACE ( 'NONE', ( #3224, #9857 ), #2245, .T. ) ;
#8983=EDGE_LOOP ( 'NONE', ( #3523, #3262, #9121, #6997 ) ) ;
#8997=ORIENTED_EDGE ( 'NONE', *, *, #8241, .T. ) ;
#8999=ORIENTED_EDGE ( 'NONE', *, *, #10767, .T. ) ;
#9003=CARTESIAN_POINT ( 'NONE',  ( -104.9999999999999289, -15.00000000000001421, -2.000000000000000000 ) ) ;
#9007=ORIENTED_EDGE ( 'NONE', *, *, #3592, .F. ) ;
#9010=VECTOR ( 'NONE', #6988, 1000.000000000000000 ) ;
#9012=ORIENTED_EDGE ( 'NONE', *, *, #5754, .F. ) ;
#9019=CARTESIAN_POINT ( 'NONE',  ( -49.99999999999998579, -15.00000000000001243, -2.000000000000000000 ) ) ;
#9041=VECTOR ( 'NONE', #6056, 1000.000000000000000 ) ;
#9047=ADVANCED_FACE ( 'NONE', ( #10894 ), #3284, .F. ) ;
#9048=DIRECTION ( 'NONE',  ( 0.000000000000000000, 0.000000000000000000, 1.000000000000000000 ) ) ;
#9049=AXIS2_PLACEMENT_3D ( 'NONE', #1297, #5443, #1120 ) ;
#9052=EDGE_CURVE ( 'NONE', #6336, #40, #4010, .T. ) ;
#9057=CARTESIAN_POINT ( 'NONE',  ( 0.000000000000000000, 0.000000000000000000, 0.000000000000000000 ) ) ;
#9061=DIRECTION ( 'NONE',  ( -0.000000000000000000, -0.000000000000000000, -1.000000000000000000 ) ) ;
#9070=CARTESIAN_POINT ( 'NONE',  ( -77.99999999999998579, -11.50000000000000711, -2.000000000000001332 ) ) ;
#9098=EDGE_CURVE ( 'NONE', #3792, #9204, #4730, .T. ) ;
#9104=AXIS2_PLACEMENT_3D ( 'NONE', #1790, #8568, #7737 ) ;
#9111=PLANE ( 'NONE',  #7078 ) ;
#9121=ORIENTED_EDGE ( 'NONE', *, *, #10836, .F. ) ;
#9130=CARTESIAN_POINT ( 'NONE',  ( -149.9999999999999716, 8.000000000000000000, 0.000000000000000000 ) ) ;
#9133=ORIENTED_EDGE ( 'NONE', *, *, #5007, .T. ) ;
#9149=CARTESIAN_POINT ( 'NONE',  ( -114.9999999999999147, -43.00000000000000000, 0.000000000000000000 ) ) ;
#9168=ORIENTED_EDGE ( 'NONE', *, *, #9950, .T. ) ;
#9170=ORIENTED_EDGE ( 'NONE', *, *, #6868, .T. ) ;
#9185=ORIENTED_EDGE ( 'NONE', *, *, #4732, .F. ) ;
#9200=VECTOR ( 'NONE', #8178, 1000.000000000000000 ) ;
#9204=VERTEX_POINT ( 'NONE', #5890 ) ;
#9208=LINE ( 'NONE', #1595, #8680 ) ;
#9212=AXIS2_PLACEMENT_3D ( 'NONE', #1230, #6114, #3665 ) ;
#9215=ORIENTED_EDGE ( 'NONE', *, *, #9484, .F. ) ;
#9241=ORIENTED_EDGE ( 'NONE', *, *, #10731, .F. ) ;
#9263=VERTEX_POINT ( 'NONE', #1947 ) ;
#9267=EDGE_CURVE ( 'NONE', #8912, #3585, #8901, .T. ) ;
#9277=CARTESIAN_POINT ( 'NONE',  ( -77.99999999999998579, -11.50000000000000711, -2.000000000000000000 ) ) ;
#9295=CARTESIAN_POINT ( 'NONE',  ( -109.9999999999999432, 14.99999999999998579, 0.000000000000000000 ) ) ;
#9306=VERTEX_POINT ( 'NONE', #7230 ) ;
#9307=CYLINDRICAL_SURFACE ( 'NONE', #4308, 1.099999999999989875 ) ;
#9312=ORIENTED_EDGE ( 'NONE', *, *, #6704, .F. ) ;
#9322=EDGE_LOOP ( 'NONE', ( #4036, #6244, #9597, #8639, #5325, #1092, #10480, #6413, #6175, #9685, #2484, #8926, #8753, #1357, #9796, #1828 ) ) ;
#9324=ORIENTED_EDGE ( 'NONE', *, *, #1644, .F. ) ;
#9340=EDGE_CURVE ( 'NONE', #8859, #3792, #4436, .T. ) ;
#9351=LINE ( 'NONE', #853, #10513 ) ;
#9368=VECTOR ( 'NONE', #7727, 1000.000000000000000 ) ;
#9372=CARTESIAN_POINT ( 'NONE',  ( -49.99999999999998579, -4.000000000000019540, -2.000000000000000000 ) ) ;
#9384=DIRECTION ( 'NONE',  ( 0.000000000000000000, 1.000000000000000000, 0.000000000000000000 ) ) ;
#9389=LINE ( 'NONE', #7566, #6007 ) ;
#9411=DIRECTION ( 'NONE',  ( 0.000000000000000000, -1.000000000000000000, 0.000000000000000000 ) ) ;
#9418=VERTEX_POINT ( 'NONE', #3608 ) ;
#9431=ORIENTED_EDGE ( 'NONE', *, *, #10261, .F. ) ;
#9444=DIRECTION ( 'NONE',  ( 0.000000000000000000, -1.000000000000000000, 0.000000000000000000 ) ) ;
#9449=LINE ( 'NONE', #8621, #4416 ) ;
#9460=VECTOR ( 'NONE', #6108, 1000.000000000000000 ) ;
#9461=EDGE_CURVE ( 'NONE', #10821, #4361, #8072, .T. ) ;
#9468=DIRECTION ( 'NONE',  ( 0.000000000000000000, 0.000000000000000000, -1.000000000000000000 ) ) ;
#9470=EDGE_LOOP ( 'NONE', ( #10124, #3887, #10824, #4096, #8962, #8847 ) ) ;
#9476=ORIENTED_EDGE ( 'NONE', *, *, #2693, .T. ) ;
#9480=ADVANCED_FACE ( 'NONE', ( #8179, #7394 ), #9111, .T. ) ;
#9484=EDGE_CURVE ( 'NONE', #7385, #3291, #719, .T. ) ;
#9498=DIRECTION ( 'NONE',  ( 1.110223024625156343E-15, 1.000000000000000000, -0.000000000000000000 ) ) ;
#9499=DIRECTION ( 'NONE',  ( 0.000000000000000000, -0.000000000000000000, -1.000000000000000000 ) ) ;
#9509=EDGE_CURVE ( 'NONE', #930, #10486, #2999, .T. ) ;
#9516=DIRECTION ( 'NONE',  ( -0.000000000000000000, -0.000000000000000000, 1.000000000000000000 ) ) ;
#9540=DIRECTION ( 'NONE',  ( 1.000000000000000000, 0.000000000000000000, 0.000000000000000000 ) ) ;
#9545=CARTESIAN_POINT ( 'NONE',  ( -57.99999999999998579, 0.000000000000000000, 0.000000000000000000 ) ) ;
#9546=CIRCLE ( 'NONE', #7265, 1.100000000000003642 ) ;
#9556=VECTOR ( 'NONE', #4498, 1000.000000000000000 ) ;
#9559=CARTESIAN_POINT ( 'NONE',  ( -57.99999999999998579, 0.000000000000000000, 3.141811147483251965 ) ) ;
#9575=CIRCLE ( 'NONE', #9049, 1.100000000000003642 ) ;
#9577=CARTESIAN_POINT ( 'NONE',  ( -120.0000000000000000, 3.999999999999980904, 0.000000000000000000 ) ) ;
#9594=CARTESIAN_POINT ( 'NONE',  ( -120.0000000000000000, 15.67949192431120053, -2.000000000000000000 ) ) ;
#9597=ORIENTED_EDGE ( 'NONE', *, *, #9894, .F. ) ;
#9599=DIRECTION ( 'NONE',  ( 0.000000000000000000, 0.000000000000000000, 1.000000000000000000 ) ) ;
#9602=CARTESIAN_POINT ( 'NONE',  ( -105.0000000000000000, -2.500000000000000000, 4.000000000000000000 ) ) ;
#9653=VERTEX_POINT ( 'NONE', #9372 ) ;
#9679=PLANE ( 'NONE',  #2840 ) ;
#9685=ORIENTED_EDGE ( 'NONE', *, *, #9844, .T. ) ;
#9694=PLANE ( 'NONE',  #1112 ) ;
#9705=LINE ( 'NONE', #8934, #3890 ) ;
#9709=LINE ( 'NONE', #5475, #5255 ) ;
#9735=VECTOR ( 'NONE', #9843, 1000.000000000000000 ) ;
#9743=CYLINDRICAL_SURFACE ( 'NONE', #2991, 1.000000000000000888 ) ;
#9745=VECTOR ( 'NONE', #10503, 1000.000000000000000 ) ;
#9767=EDGE_LOOP ( 'NONE', ( #2110, #8184 ) ) ;
#9774=EDGE_LOOP ( 'NONE', ( #7273, #9851, #2826, #7891 ) ) ;
#9776=DIRECTION ( 'NONE',  ( 0.000000000000000000, 1.000000000000000000, 0.000000000000000000 ) ) ;
#9783=CARTESIAN_POINT ( 'NONE',  ( -49.99999999999998579, 2.500000000000000000, 3.000000000000000000 ) ) ;
#9796=ORIENTED_EDGE ( 'NONE', *, *, #10843, .F. ) ;
#9804=CARTESIAN_POINT ( 'NONE',  ( -49.99998799999998766, 0.000000000000000000, 3.141811147483251965 ) ) ;
#9807=EDGE_LOOP ( 'NONE', ( #4083, #2171, #7244, #2865 ) ) ;
#9809=VECTOR ( 'NONE', #4003, 1000.000000000000000 ) ;
#9817=PLANE ( 'NONE',  #5893 ) ;
#9834=DIRECTION ( 'NONE',  ( 0.000000000000000000, 0.000000000000000000, -1.000000000000000000 ) ) ;
#9843=DIRECTION ( 'NONE',  ( -1.000000000000000000, -0.000000000000000000, -0.000000000000000000 ) ) ;
#9844=EDGE_CURVE ( 'NONE', #211, #9653, #4596, .T. ) ;
#9849=CARTESIAN_POINT ( 'NONE',  ( -120.0000000000000000, 14.99999999999998579, -2.000000000000000000 ) ) ;
#9851=ORIENTED_EDGE ( 'NONE', *, *, #8536, .F. ) ;
#9857=FACE_OUTER_BOUND ( 'NONE', #10663, .T. ) ;
#9859=EDGE_CURVE ( 'NONE', #6336, #10601, #208, .T. ) ;
#9864=CARTESIAN_POINT ( 'NONE',  ( -120.0000000000000000, 14.99999999999998579, 83.15773105863907233 ) ) ;
#9873=ADVANCED_FACE ( 'NONE', ( #1275 ), #152, .F. ) ;
#9884=ORIENTED_EDGE ( 'NONE', *, *, #10767, .F. ) ;
#9885=CARTESIAN_POINT ( 'NONE',  ( -61.99999999999998579, -15.00000000000001421, 0.5000000000000013323 ) ) ;
#9894=EDGE_CURVE ( 'NONE', #4539, #7385, #10426, .T. ) ;
#9895=CARTESIAN_POINT ( 'NONE',  ( -114.9999999999999147, -43.00000000000000000, 0.000000000000000000 ) ) ;
#9902=LINE ( 'NONE', #1459, #1474 ) ;
#9917=CARTESIAN_POINT ( 'NONE',  ( -120.0000000000000000, 3.999999999999980904, 0.000000000000000000 ) ) ;
#9924=ORIENTED_EDGE ( 'NONE', *, *, #4446, .F. ) ;
#9928=AXIS2_PLACEMENT_3D ( 'NONE', #7009, #2067, #9499 ) ;
#9930=VECTOR ( 'NONE', #2935, 1000.000000000000000 ) ;
#9950=EDGE_CURVE ( 'NONE', #2208, #7538, #6368, .T. ) ;
#9953=LINE ( 'NONE', #9895, #9809 ) ;
#9959=EDGE_CURVE ( 'NONE', #1714, #5618, #7259, .T. ) ;
#9961=DIRECTION ( 'NONE',  ( -0.000000000000000000, -0.000000000000000000, 1.000000000000000000 ) ) ;
#9968=EDGE_LOOP ( 'NONE', ( #7398, #1918, #880, #865 ) ) ;
#9970=CARTESIAN_POINT ( 'NONE',  ( -57.99999999999998579, -14.00000000000001243, 0.000000000000000000 ) ) ;
#9986=VECTOR ( 'NONE', #324, 1000.000000000000000 ) ;
#9987=CIRCLE ( 'NONE', #8049, 20.00000000000000355 ) ;
#9999=EDGE_CURVE ( 'NONE', #7538, #930, #6608, .T. ) ;
#10009=DIRECTION ( 'NONE',  ( -0.000000000000000000, -0.000000000000000000, -1.000000000000000000 ) ) ;
#10014=CARTESIAN_POINT ( 'NONE',  ( -61.99999999999998579, -8.000000000000000000, 2.500000000000003109 ) ) ;
#10027=EDGE_CURVE ( 'NONE', #4585, #3431, #498, .T. ) ;
#10029=CARTESIAN_POINT ( 'NONE',  ( 0.000000000000000000, 0.000000000000000000, 0.000000000000000000 ) ) ;
#10032=( NAMED_UNIT ( * ) SI_UNIT ( $, .STERADIAN. ) SOLID_ANGLE_UNIT ( ) );
#10045=UNCERTAINTY_MEASURE_WITH_UNIT (LENGTH_MEASURE( 1.000000000000000082E-05 ), #6328, 'distance_accuracy_value', 'NONE');
#10055=DIRECTION ( 'NONE',  ( 0.000000000000000000, 1.000000000000000000, 0.000000000000000000 ) ) ;
#10074=PLANE ( 'NONE',  #2352 ) ;
#10078=DIRECTION ( 'NONE',  ( -0.000000000000000000, -0.000000000000000000, 1.000000000000000000 ) ) ;
#10079=EDGE_LOOP ( 'NONE', ( #4460, #9215, #1042, #3396, #1602, #3014, #10567, #4516, #4593 ) ) ;
#10085=DIRECTION ( 'NONE',  ( 0.000000000000000000, -0.000000000000000000, 1.000000000000000000 ) ) ;
#10095=VECTOR ( 'NONE', #1355, 1000.000000000000000 ) ;
#10099=LINE ( 'NONE', #4967, #10861 ) ;
#10103=CARTESIAN_POINT ( 'NONE',  ( -61.99999999999998579, 8.000000000000000000, 1.500000000000002220 ) ) ;
#10124=ORIENTED_EDGE ( 'NONE', *, *, #7226, .F. ) ;
#10135=ORIENTED_EDGE ( 'NONE', *, *, #10589, .T. ) ;
#10137=ORIENTED_EDGE ( 'NONE', *, *, #10310, .F. ) ;
#10141=ORIENTED_EDGE ( 'NONE', *, *, #6545, .F. ) ;
#10146=VECTOR ( 'NONE', #8410, 1000.000000000000000 ) ;
#10162=LINE ( 'NONE', #2560, #6900 ) ;
#10168=CARTESIAN_POINT ( 'NONE',  ( -120.0000000000000000, -15.00000000000001421, 5.000000000000004441 ) ) ;
#10181=FACE_OUTER_BOUND ( 'NONE', #1370, .T. ) ;
#10184=EDGE_CURVE ( 'NONE', #5900, #4466, #1756, .T. ) ;
#10185=EDGE_LOOP ( 'NONE', ( #4300, #5827, #8869, #3257 ) ) ;
#10186=CARTESIAN_POINT ( 'NONE',  ( -77.99999999999998579, -11.50000000000000711, -2.000000000000001332 ) ) ;
#10192=CARTESIAN_POINT ( 'NONE',  ( -49.99999999999998579, 3.999999999999980904, -2.000000000000000000 ) ) ;
#10201=EDGE_LOOP ( 'NONE', ( #2625, #5979, #7182, #5533 ) ) ;
#10207=LINE ( 'NONE', #5995, #1923 ) ;
#10212=CARTESIAN_POINT ( 'NONE',  ( -49.99999999999998579, -8.000000000000000000, 83.15773105863907233 ) ) ;
#10232=VECTOR ( 'NONE', #10078, 1000.000000000000000 ) ;
#10236=EDGE_LOOP ( 'NONE', ( #2399, #6418, #6237, #6606 ) ) ;
#10253=VECTOR ( 'NONE', #10561, 1000.000000000000000 ) ;
#10261=EDGE_CURVE ( 'NONE', #6858, #6924, #2418, .T. ) ;
#10263=AXIS2_PLACEMENT_3D ( 'NONE', #3586, #10305, #6932 ) ;
#10299=SURFACE_STYLE_FILL_AREA ( #137 ) ;
#10305=DIRECTION ( 'NONE',  ( -2.478176394252581696E-17, 1.000000000000000000, 0.000000000000000000 ) ) ;
#10310=EDGE_CURVE ( 'NONE', #8229, #10601, #6144, .T. ) ;
#10315=ORIENTED_EDGE ( 'NONE', *, *, #2401, .F. ) ;
#10317=DIRECTION ( 'NONE',  ( 1.000000000000000000, 0.000000000000000000, 0.000000000000000000 ) ) ;
#10376=ADVANCED_FACE ( 'NONE', ( #1082 ), #310, .T. ) ;
#10377=APPLICATION_CONTEXT ( 'automotive_design' ) ;
#10378=EDGE_LOOP ( 'NONE', ( #7335, #2650, #9476, #9007 ) ) ;
#10392=DIRECTION ( 'NONE',  ( -0.000000000000000000, -1.000000000000000000, -0.000000000000000000 ) ) ;
#10396=DIRECTION ( 'NONE',  ( -0.000000000000000000, 1.000000000000000000, -0.000000000000000000 ) ) ;
#10410=ORIENTED_EDGE ( 'NONE', *, *, #6658, .F. ) ;
#10426=LINE ( 'NONE', #2829, #1214 ) ;
#10428=DIRECTION ( 'NONE',  ( -1.000000000000000000, 8.673617379884033500E-16, 0.000000000000000000 ) ) ;
#10431=AXIS2_PLACEMENT_3D ( 'NONE', #4983, #4929, #8384 ) ;
#10433=VERTEX_POINT ( 'NONE', #4347 ) ;
#10437=CARTESIAN_POINT ( 'NONE',  ( -57.99999999999998579, 0.000000000000000000, -0.1418111474832477736 ) ) ;
#10440=EDGE_CURVE ( 'NONE', #8694, #4585, #6983, .T. ) ;
#10463=CARTESIAN_POINT ( 'NONE',  ( -114.9999999999999147, -43.00000000000000000, -2.000000000000000000 ) ) ;
#10470=LINE ( 'NONE', #10585, #4815 ) ;
#10480=ORIENTED_EDGE ( 'NONE', *, *, #5529, .F. ) ;
#10486=VERTEX_POINT ( 'NONE', #7465 ) ;
#10490=LINE ( 'NONE', #2053, #6446 ) ;
#10500=EDGE_CURVE ( 'NONE', #4198, #544, #6321, .T. ) ;
#10503=DIRECTION ( 'NONE',  ( -0.000000000000000000, -0.000000000000000000, 1.000000000000000000 ) ) ;
#10513=VECTOR ( 'NONE', #2366, 1000.000000000000000 ) ;
#10516=AXIS2_PLACEMENT_3D ( 'NONE', #616, #4768, #8276 ) ;
#10533=VECTOR ( 'NONE', #9516, 1000.000000000000000 ) ;
#10536=CARTESIAN_POINT ( 'NONE',  ( -120.0000000000000000, -15.00000000000001421, -2.000000000000000000 ) ) ;
#10550=CARTESIAN_POINT ( 'NONE',  ( -120.0000000000000000, -15.00000000000001421, -2.000000000000000000 ) ) ;
#10553=ORIENTED_EDGE ( 'NONE', *, *, #851, .F. ) ;
#10554=DIRECTION ( 'NONE',  ( 0.000000000000000000, 1.000000000000000000, -5.282956808509869699E-16 ) ) ;
#10561=DIRECTION ( 'NONE',  ( -0.000000000000000000, 1.000000000000000000, -0.000000000000000000 ) ) ;
#10564=ORIENTED_EDGE ( 'NONE', *, *, #5591, .T. ) ;
#10566=CARTESIAN_POINT ( 'NONE',  ( -49.99999999999998579, -15.00000000000001243, 83.15773105863907233 ) ) ;
#10567=ORIENTED_EDGE ( 'NONE', *, *, #8744, .T. ) ;
#10582=ORIENTED_EDGE ( 'NONE', *, *, #7753, .T. ) ;
#10585=CARTESIAN_POINT ( 'NONE',  ( -49.99999999999998579, -10.00000000000000888, 83.15773105863907233 ) ) ;
#10589=EDGE_CURVE ( 'NONE', #8768, #8566, #9705, .T. ) ;
#10601=VERTEX_POINT ( 'NONE', #734 ) ;
#10604=VECTOR ( 'NONE', #9468, 1000.000000000000000 ) ;
#10609=DIRECTION ( 'NONE',  ( -1.000000000000000000, 0.000000000000000000, -0.000000000000000000 ) ) ;
#10620=EDGE_CURVE ( 'NONE', #4626, #2204, #8351, .T. ) ;
#10642=ORIENTED_EDGE ( 'NONE', *, *, #5576, .T. ) ;
#10658=ORIENTED_EDGE ( 'NONE', *, *, #6274, .F. ) ;
#10663=EDGE_LOOP ( 'NONE', ( #2665, #6105, #10137, #5819, #9241, #6047 ) ) ;
#10664=LINE ( 'NONE', #4870, #7109 ) ;
#10666=ORIENTED_EDGE ( 'NONE', *, *, #7333, .T. ) ;
#10680=DIRECTION ( 'NONE',  ( 0.000000000000000000, 0.000000000000000000, 1.000000000000000000 ) ) ;
#10681=EDGE_CURVE ( 'NONE', #3104, #3152, #10162, .T. ) ;
#10682=ORIENTED_EDGE ( 'NONE', *, *, #572, .F. ) ;
#10691=FACE_OUTER_BOUND ( 'NONE', #10201, .T. ) ;
#10719=CARTESIAN_POINT ( 'NONE',  ( -61.99999999999998579, -8.000000000000000000, 1.500000000000002220 ) ) ;
#10720=AXIS2_PLACEMENT_3D ( 'NONE', #10186, #9061, #8425 ) ;
#10725=PLANE ( 'NONE',  #8227 ) ;
#10731=EDGE_CURVE ( 'NONE', #2188, #5900, #1725, .T. ) ;
#10735=DIRECTION ( 'NONE',  ( 1.110223024625156343E-15, 1.000000000000000000, -0.000000000000000000 ) ) ;
#10736=LINE ( 'NONE', #5672, #8580 ) ;
#10749=DIRECTION ( 'NONE',  ( 0.000000000000000000, -1.000000000000000000, 0.000000000000000000 ) ) ;
#10753=ORIENTED_EDGE ( 'NONE', *, *, #6274, .T. ) ;
#10767=EDGE_CURVE ( 'NONE', #8768, #3366, #3495, .T. ) ;
#10769=CARTESIAN_POINT ( 'NONE',  ( -109.9999999999999289, 33.00000000000000711, -2.000000000000000000 ) ) ;
#10794=VECTOR ( 'NONE', #5435, 1000.000000000000000 ) ;
#10803=DIRECTION ( 'NONE',  ( -3.469446951953572774E-16, 1.000000000000000000, 0.000000000000000000 ) ) ;
#10809=DIRECTION ( 'NONE',  ( -1.000000000000000000, 0.000000000000000000, 0.000000000000000000 ) ) ;
#10812=VECTOR ( 'NONE', #6005, 1000.000000000000000 ) ;
#10813=EDGE_CURVE ( 'NONE', #7749, #3994, #5155, .T. ) ;
#10814=EDGE_LOOP ( 'NONE', ( #10975, #9324 ) ) ;
#10815=MECHANICAL_DESIGN_GEOMETRIC_PRESENTATION_REPRESENTATION('',(#1765),#6206);
#10820=CARTESIAN_POINT ( 'NONE',  ( -49.99999999999998579, -15.00000000000001243, 3.000000000000002665 ) ) ;
#10821=VERTEX_POINT ( 'NONE', #5999 ) ;
#10824=ORIENTED_EDGE ( 'NONE', *, *, #3592, .T. ) ;
#10825=DIRECTION ( 'NONE',  ( 1.000000000000000000, -1.110223024625156343E-15, 0.000000000000000000 ) ) ;
#10834=DIRECTION ( 'NONE',  ( 0.000000000000000000, -0.000000000000000000, 1.000000000000000000 ) ) ;
#10836=EDGE_CURVE ( 'NONE', #4938, #9653, #2676, .T. ) ;
#10843=EDGE_CURVE ( 'NONE', #3152, #544, #4374, .T. ) ;
#10846=DIRECTION ( 'NONE',  ( 1.000000000000000000, 0.000000000000000000, -0.000000000000000000 ) ) ;
#10850=DIRECTION ( 'NONE',  ( 0.000000000000000000, 0.000000000000000000, -1.000000000000000000 ) ) ;
#10851=DIRECTION ( 'NONE',  ( 0.000000000000000000, 0.000000000000000000, 1.000000000000000000 ) ) ;
#10852=CIRCLE ( 'NONE', #6059, 1.100000000000003642 ) ;
#10861=VECTOR ( 'NONE', #3375, 1000.000000000000000 ) ;
#10866=EDGE_LOOP ( 'NONE', ( #2092, #527, #8938, #6550 ) ) ;
#10874=VECTOR ( 'NONE', #2747, 1000.000000000000000 ) ;
#10877=PLANE ( 'NONE',  #1623 ) ;
#10878=EDGE_CURVE ( 'NONE', #6336, #10433, #7123, .T. ) ;
#10882=VECTOR ( 'NONE', #7338, 1000.000000000000000 ) ;
#10887=DIRECTION ( 'NONE',  ( 0.000000000000000000, -5.282956808509868713E-16, -1.000000000000000000 ) ) ;
#10894=FACE_OUTER_BOUND ( 'NONE', #5068, .T. ) ;
#10898=DIRECTION ( 'NONE',  ( 0.000000000000000000, -1.000000000000000000, 0.000000000000000000 ) ) ;
#10909=ORIENTED_EDGE ( 'NONE', *, *, #1987, .F. ) ;
#10962=ORIENTED_EDGE ( 'NONE', *, *, #8078, .T. ) ;
#10964=AXIS2_PLACEMENT_3D ( 'NONE', #10719, #9776, #9048 ) ;
#10974=VECTOR ( 'NONE', #9498, 1000.000000000000000 ) ;
#10975=ORIENTED_EDGE ( 'NONE', *, *, #1748, .F. ) ;
#10976=CARTESIAN_POINT ( 'NONE',  ( -120.0000000000000000, -15.00000000000001421, 0.000000000000000000 ) ) ;
#11007=COLOUR_RGB('Sky Blue',0.24,0.69,0.87);
#11008=FILL_AREA_STYLE_COLOUR('',#11007);
#11009=FILL_AREA_STYLE('',(#11008));
#11010=SURFACE_STYLE_FILL_AREA(#11009);
#11011=SURFACE_SIDE_STYLE('',(#11010));
#11012=SURFACE_STYLE_USAGE(.BOTH.,#11011);
#11013=PRESENTATION_STYLE_ASSIGNMENT((#11012));
ENDSEC;
END-ISO-10303-21;
